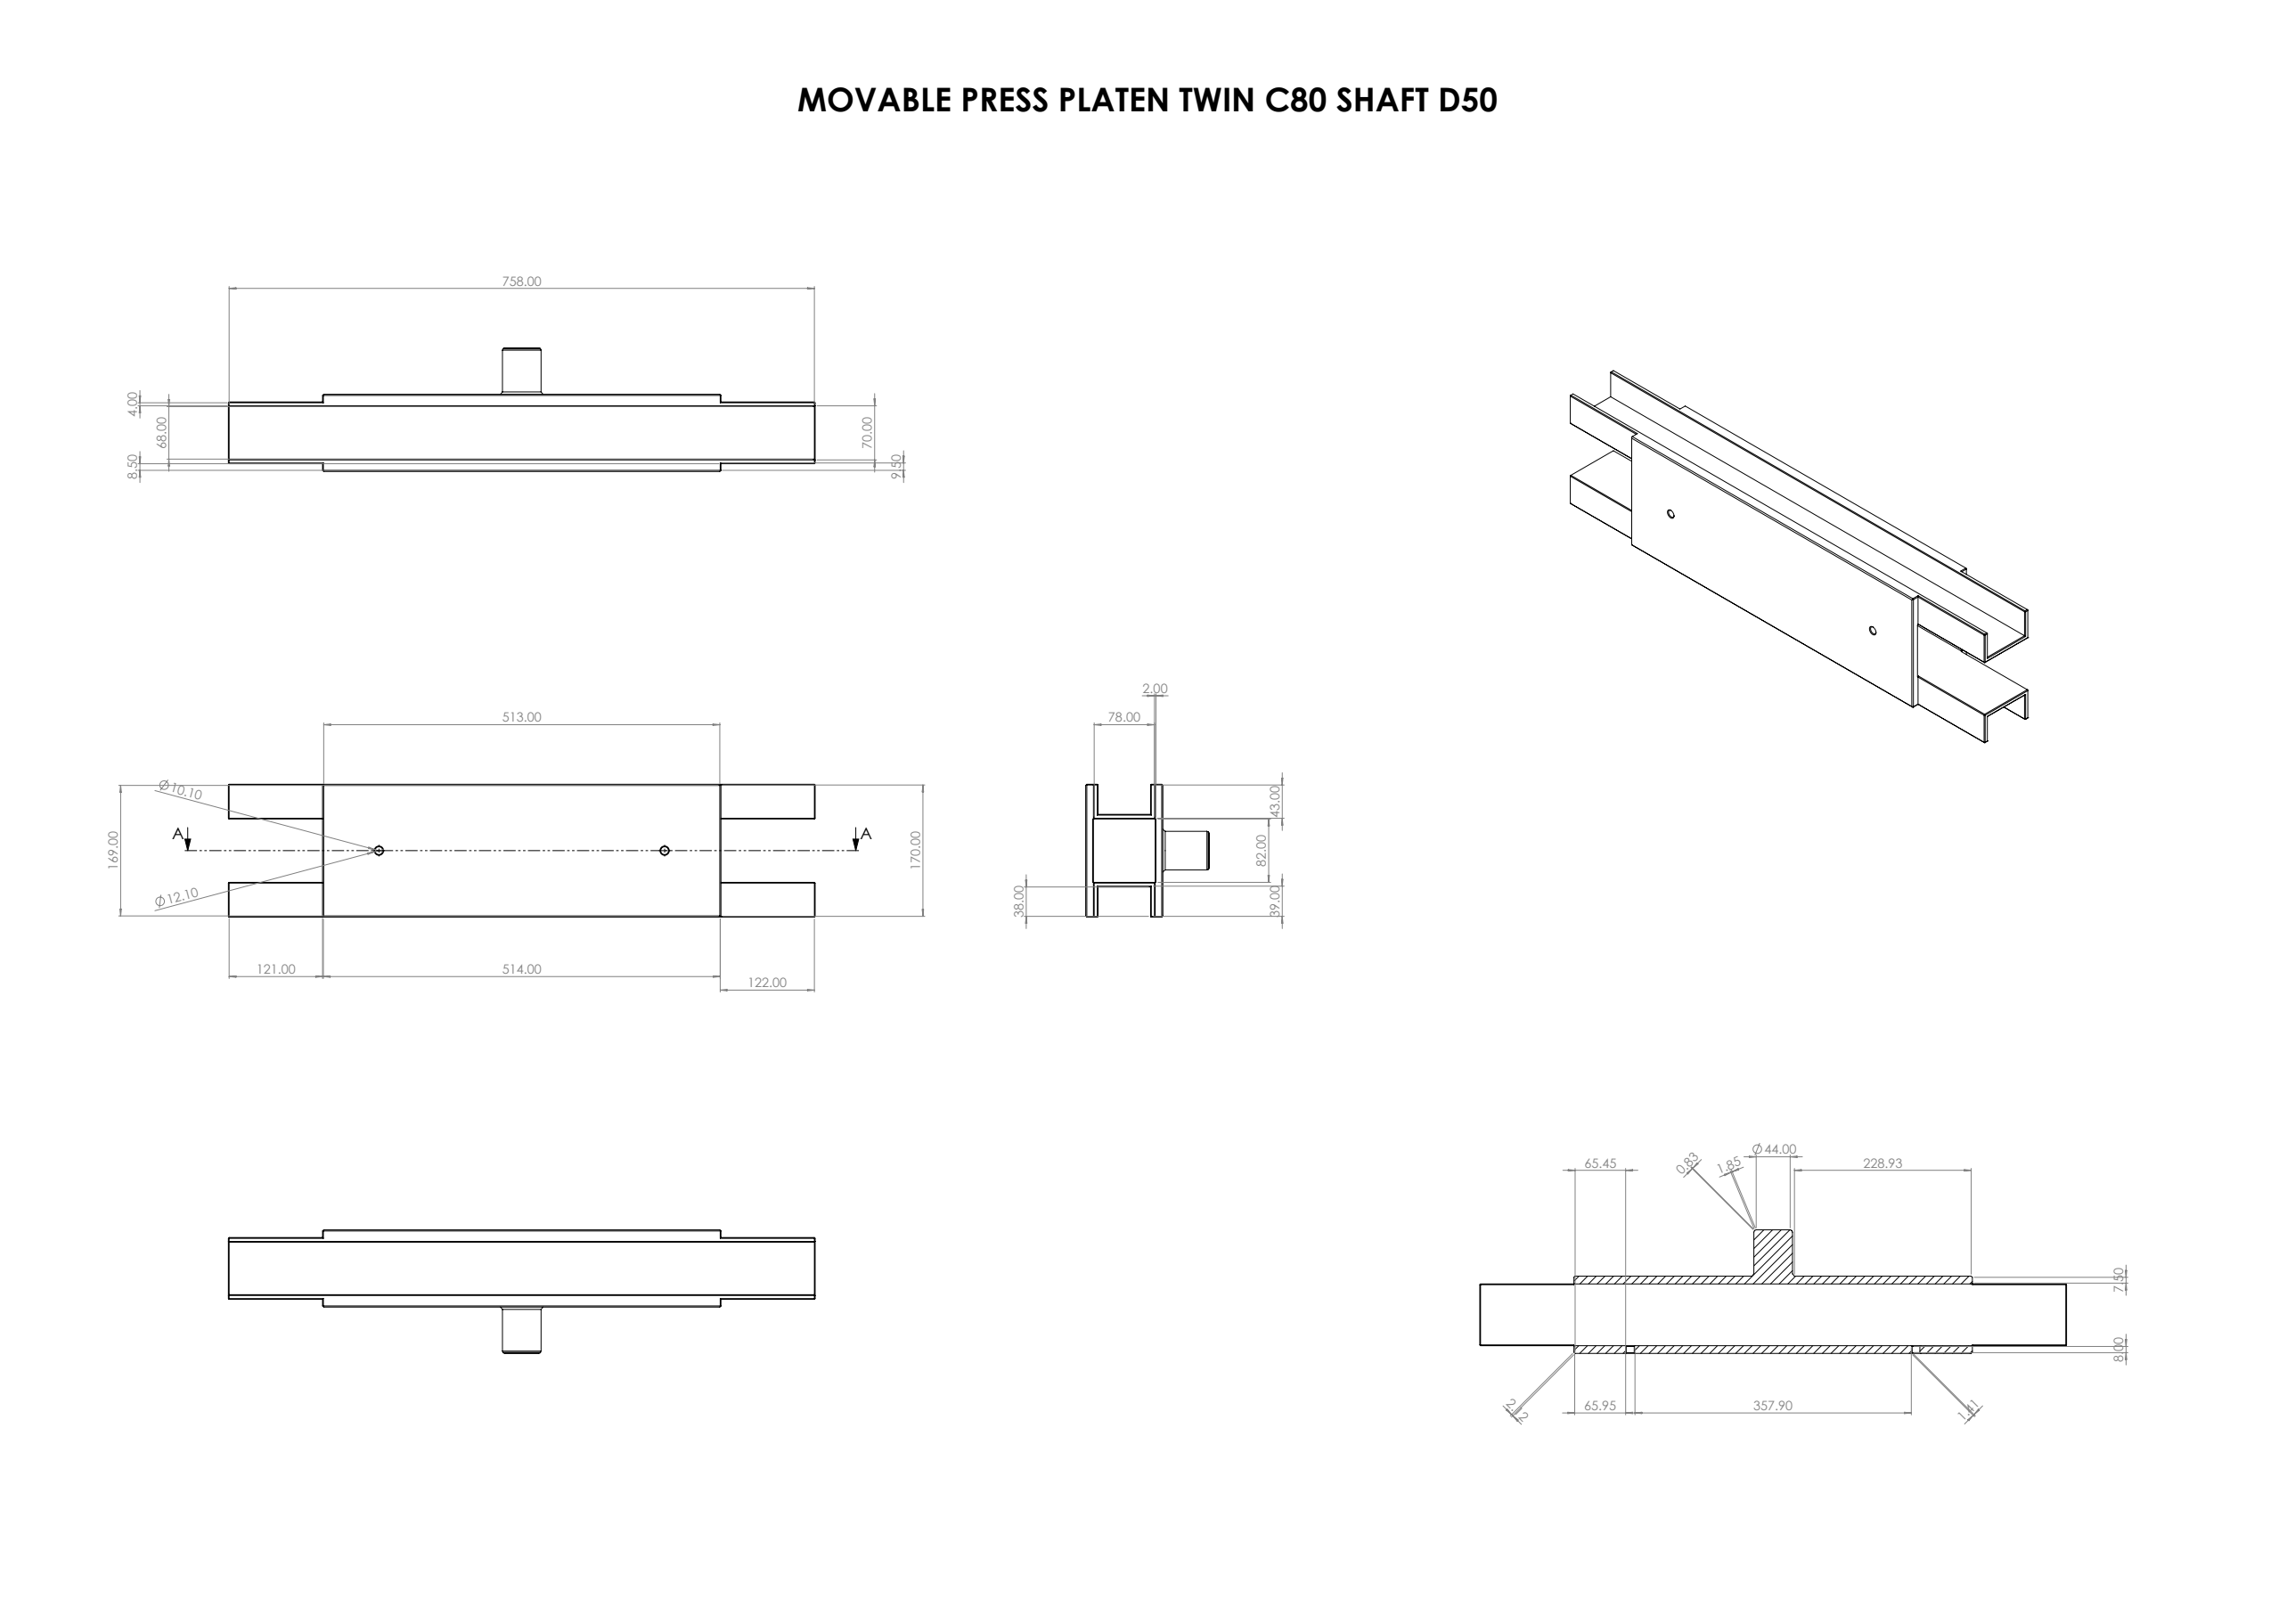
ISO-10303-21;
HEADER;
/* Generated by software containing ST-Developer
 * from STEP Tools, Inc. (www.steptools.com) 
 */

FILE_DESCRIPTION(
/* description */ (''),
/* implementation_level */ '2;1');

FILE_NAME(
/* name */ '03_Movable_Press_Platen_Twin_C80_Shaft_D50.step',
/* time_stamp */ '2026-10-20T10:03:03-07:00',
/* author */ (''),
/* organization */ (''),
/* preprocessor_version */ 'ST-DEVELOPER v20.2',
/* originating_system */ 'Autodesk Translation Framework v15.15.0.0',
/* authorisation */ '');

FILE_SCHEMA (('AUTOMOTIVE_DESIGN { 1 0 10303 214 3 1 1 }'));
ENDSEC;

DATA;
#10=MECHANICAL_DESIGN_GEOMETRIC_PRESENTATION_REPRESENTATION('',(#525),#71492);
#383=SHAPE_REPRESENTATION_RELATIONSHIP('SRR','None',#71604,#402);
#402=ADVANCED_BREP_SHAPE_REPRESENTATION('',(#421),#71474);
#421=MANIFOLD_SOLID_BREP('Platen',#28460);
#525=STYLED_ITEM('',(#71887),#421);
#1566=CYLINDRICAL_SURFACE('',#29155,2.5);
#1567=CYLINDRICAL_SURFACE('',#29162,0.504999999999999);
#1568=CYLINDRICAL_SURFACE('',#29170,0.504999999999999);
#1905=FACE_BOUND('',#4962,.T.);
#1906=FACE_BOUND('',#4963,.T.);
#1907=FACE_BOUND('',#5001,.T.);
#1908=FACE_BOUND('',#5002,.T.);
#1909=FACE_BOUND('',#5010,.T.);
#2197=CIRCLE('',#29117,0.605);
#2198=CIRCLE('',#29118,0.605);
#2199=CIRCLE('',#29148,2.5);
#2200=CIRCLE('',#29149,2.5);
#2201=CIRCLE('',#29150,2.42928932188135);
#2202=CIRCLE('',#29151,2.42928932188135);
#2203=CIRCLE('',#29153,2.37071067811866);
#2204=CIRCLE('',#29154,2.37071067811866);
#2205=CIRCLE('',#29156,2.5);
#2206=CIRCLE('',#29158,2.2);
#2207=CIRCLE('',#29161,0.504999999999999);
#2208=CIRCLE('',#29163,0.504999999999999);
#2209=CIRCLE('',#29165,0.605);
#2210=CIRCLE('',#29167,0.605);
#2211=CIRCLE('',#29169,0.504999999999999);
#2212=CIRCLE('',#29171,0.504999999999999);
#2213=CIRCLE('',#29174,2.75714285714286);
#2799=CONICAL_SURFACE('',#29147,2.46464466094067,0.392699081698708);
#2800=CONICAL_SURFACE('',#29152,2.4,0.785398163397442);
#2801=CONICAL_SURFACE('',#29157,2.28535533905933,1.17809724509617);
#2802=CONICAL_SURFACE('',#29160,0.555,0.785398163397484);
#2803=CONICAL_SURFACE('',#29164,0.555,0.785398163397484);
#2804=CONICAL_SURFACE('',#29168,0.555,0.785398163397484);
#2805=CONICAL_SURFACE('',#29172,0.555,0.785398163397484);
#2806=CONICAL_SURFACE('',#29173,2.65,0.708626272127678);
#3280=FACE_OUTER_BOUND('',#4891,.T.);
#3281=FACE_OUTER_BOUND('',#4892,.T.);
#3282=FACE_OUTER_BOUND('',#4893,.T.);
#3283=FACE_OUTER_BOUND('',#4894,.T.);
#3284=FACE_OUTER_BOUND('',#4895,.T.);
#3285=FACE_OUTER_BOUND('',#4896,.T.);
#3286=FACE_OUTER_BOUND('',#4897,.T.);
#3287=FACE_OUTER_BOUND('',#4898,.T.);
#3288=FACE_OUTER_BOUND('',#4899,.T.);
#3289=FACE_OUTER_BOUND('',#4900,.T.);
#3290=FACE_OUTER_BOUND('',#4901,.T.);
#3291=FACE_OUTER_BOUND('',#4902,.T.);
#3292=FACE_OUTER_BOUND('',#4903,.T.);
#3293=FACE_OUTER_BOUND('',#4904,.T.);
#3294=FACE_OUTER_BOUND('',#4905,.T.);
#3295=FACE_OUTER_BOUND('',#4906,.T.);
#3296=FACE_OUTER_BOUND('',#4907,.T.);
#3297=FACE_OUTER_BOUND('',#4908,.T.);
#3298=FACE_OUTER_BOUND('',#4909,.T.);
#3299=FACE_OUTER_BOUND('',#4910,.T.);
#3300=FACE_OUTER_BOUND('',#4911,.T.);
#3301=FACE_OUTER_BOUND('',#4912,.T.);
#3302=FACE_OUTER_BOUND('',#4913,.T.);
#3303=FACE_OUTER_BOUND('',#4914,.T.);
#3304=FACE_OUTER_BOUND('',#4915,.T.);
#3305=FACE_OUTER_BOUND('',#4916,.T.);
#3306=FACE_OUTER_BOUND('',#4917,.T.);
#3307=FACE_OUTER_BOUND('',#4918,.T.);
#3308=FACE_OUTER_BOUND('',#4919,.T.);
#3309=FACE_OUTER_BOUND('',#4920,.T.);
#3310=FACE_OUTER_BOUND('',#4921,.T.);
#3311=FACE_OUTER_BOUND('',#4922,.T.);
#3312=FACE_OUTER_BOUND('',#4923,.T.);
#3313=FACE_OUTER_BOUND('',#4924,.T.);
#3314=FACE_OUTER_BOUND('',#4925,.T.);
#3315=FACE_OUTER_BOUND('',#4926,.T.);
#3316=FACE_OUTER_BOUND('',#4927,.T.);
#3317=FACE_OUTER_BOUND('',#4928,.T.);
#3318=FACE_OUTER_BOUND('',#4929,.T.);
#3319=FACE_OUTER_BOUND('',#4930,.T.);
#3320=FACE_OUTER_BOUND('',#4931,.T.);
#3321=FACE_OUTER_BOUND('',#4932,.T.);
#3322=FACE_OUTER_BOUND('',#4933,.T.);
#3323=FACE_OUTER_BOUND('',#4934,.T.);
#3324=FACE_OUTER_BOUND('',#4935,.T.);
#3325=FACE_OUTER_BOUND('',#4936,.T.);
#3326=FACE_OUTER_BOUND('',#4937,.T.);
#3327=FACE_OUTER_BOUND('',#4938,.T.);
#3328=FACE_OUTER_BOUND('',#4939,.T.);
#3329=FACE_OUTER_BOUND('',#4940,.T.);
#3330=FACE_OUTER_BOUND('',#4941,.T.);
#3331=FACE_OUTER_BOUND('',#4942,.T.);
#3332=FACE_OUTER_BOUND('',#4943,.T.);
#3333=FACE_OUTER_BOUND('',#4944,.T.);
#3334=FACE_OUTER_BOUND('',#4945,.T.);
#3335=FACE_OUTER_BOUND('',#4946,.T.);
#3336=FACE_OUTER_BOUND('',#4947,.T.);
#3337=FACE_OUTER_BOUND('',#4948,.T.);
#3338=FACE_OUTER_BOUND('',#4949,.T.);
#3339=FACE_OUTER_BOUND('',#4950,.T.);
#3340=FACE_OUTER_BOUND('',#4951,.T.);
#3341=FACE_OUTER_BOUND('',#4952,.T.);
#3342=FACE_OUTER_BOUND('',#4953,.T.);
#3343=FACE_OUTER_BOUND('',#4954,.T.);
#3344=FACE_OUTER_BOUND('',#4955,.T.);
#3345=FACE_OUTER_BOUND('',#4956,.T.);
#3346=FACE_OUTER_BOUND('',#4957,.T.);
#3347=FACE_OUTER_BOUND('',#4958,.T.);
#3348=FACE_OUTER_BOUND('',#4959,.T.);
#3349=FACE_OUTER_BOUND('',#4960,.T.);
#3350=FACE_OUTER_BOUND('',#4961,.T.);
#3351=FACE_OUTER_BOUND('',#4964,.T.);
#3352=FACE_OUTER_BOUND('',#4965,.T.);
#3353=FACE_OUTER_BOUND('',#4966,.T.);
#3354=FACE_OUTER_BOUND('',#4967,.T.);
#3355=FACE_OUTER_BOUND('',#4968,.T.);
#3356=FACE_OUTER_BOUND('',#4969,.T.);
#3357=FACE_OUTER_BOUND('',#4970,.T.);
#3358=FACE_OUTER_BOUND('',#4971,.T.);
#3359=FACE_OUTER_BOUND('',#4972,.T.);
#3360=FACE_OUTER_BOUND('',#4973,.T.);
#3361=FACE_OUTER_BOUND('',#4974,.T.);
#3362=FACE_OUTER_BOUND('',#4975,.T.);
#3363=FACE_OUTER_BOUND('',#4976,.T.);
#3364=FACE_OUTER_BOUND('',#4977,.T.);
#3365=FACE_OUTER_BOUND('',#4978,.T.);
#3366=FACE_OUTER_BOUND('',#4979,.T.);
#3367=FACE_OUTER_BOUND('',#4980,.T.);
#3368=FACE_OUTER_BOUND('',#4981,.T.);
#3369=FACE_OUTER_BOUND('',#4982,.T.);
#3370=FACE_OUTER_BOUND('',#4983,.T.);
#3371=FACE_OUTER_BOUND('',#4984,.T.);
#3372=FACE_OUTER_BOUND('',#4985,.T.);
#3373=FACE_OUTER_BOUND('',#4986,.T.);
#3374=FACE_OUTER_BOUND('',#4987,.T.);
#3375=FACE_OUTER_BOUND('',#4988,.T.);
#3376=FACE_OUTER_BOUND('',#4989,.T.);
#3377=FACE_OUTER_BOUND('',#4990,.T.);
#3378=FACE_OUTER_BOUND('',#4991,.T.);
#3379=FACE_OUTER_BOUND('',#4992,.T.);
#3380=FACE_OUTER_BOUND('',#4993,.T.);
#3381=FACE_OUTER_BOUND('',#4994,.T.);
#3382=FACE_OUTER_BOUND('',#4995,.T.);
#3383=FACE_OUTER_BOUND('',#4996,.T.);
#3384=FACE_OUTER_BOUND('',#4997,.T.);
#3385=FACE_OUTER_BOUND('',#4998,.T.);
#3386=FACE_OUTER_BOUND('',#4999,.T.);
#3387=FACE_OUTER_BOUND('',#5000,.T.);
#3388=FACE_OUTER_BOUND('',#5003,.T.);
#3389=FACE_OUTER_BOUND('',#5004,.T.);
#3390=FACE_OUTER_BOUND('',#5005,.T.);
#3391=FACE_OUTER_BOUND('',#5006,.T.);
#3392=FACE_OUTER_BOUND('',#5007,.T.);
#3393=FACE_OUTER_BOUND('',#5008,.T.);
#3394=FACE_OUTER_BOUND('',#5009,.T.);
#3395=FACE_OUTER_BOUND('',#5011,.T.);
#3396=FACE_OUTER_BOUND('',#5012,.T.);
#3397=FACE_OUTER_BOUND('',#5013,.T.);
#4891=EDGE_LOOP('',(#19603,#19604,#19605,#19606));
#4892=EDGE_LOOP('',(#19607,#19608,#19609,#19610,#19611));
#4893=EDGE_LOOP('',(#19612,#19613,#19614,#19615));
#4894=EDGE_LOOP('',(#19616,#19617,#19618,#19619));
#4895=EDGE_LOOP('',(#19620,#19621,#19622,#19623,#19624,#19625));
#4896=EDGE_LOOP('',(#19626,#19627,#19628,#19629,#19630));
#4897=EDGE_LOOP('',(#19631,#19632,#19633,#19634));
#4898=EDGE_LOOP('',(#19635,#19636,#19637,#19638,#19639));
#4899=EDGE_LOOP('',(#19640,#19641,#19642,#19643,#19644,#19645));
#4900=EDGE_LOOP('',(#19646,#19647,#19648,#19649));
#4901=EDGE_LOOP('',(#19650,#19651,#19652,#19653));
#4902=EDGE_LOOP('',(#19654,#19655,#19656,#19657));
#4903=EDGE_LOOP('',(#19658,#19659,#19660,#19661,#19662,#19663));
#4904=EDGE_LOOP('',(#19664,#19665,#19666,#19667,#19668,#19669));
#4905=EDGE_LOOP('',(#19670,#19671,#19672,#19673,#19674));
#4906=EDGE_LOOP('',(#19675,#19676,#19677,#19678,#19679,#19680));
#4907=EDGE_LOOP('',(#19681,#19682,#19683,#19684,#19685,#19686,#19687,#19688));
#4908=EDGE_LOOP('',(#19689,#19690,#19691,#19692,#19693));
#4909=EDGE_LOOP('',(#19694,#19695,#19696,#19697,#19698));
#4910=EDGE_LOOP('',(#19699,#19700,#19701,#19702,#19703,#19704,#19705,#19706));
#4911=EDGE_LOOP('',(#19707,#19708,#19709,#19710,#19711,#19712));
#4912=EDGE_LOOP('',(#19713,#19714,#19715,#19716,#19717,#19718));
#4913=EDGE_LOOP('',(#19719,#19720,#19721,#19722,#19723));
#4914=EDGE_LOOP('',(#19724,#19725,#19726,#19727,#19728,#19729));
#4915=EDGE_LOOP('',(#19730,#19731,#19732,#19733,#19734,#19735));
#4916=EDGE_LOOP('',(#19736,#19737,#19738,#19739,#19740));
#4917=EDGE_LOOP('',(#19741,#19742,#19743,#19744,#19745,#19746));
#4918=EDGE_LOOP('',(#19747,#19748,#19749,#19750,#19751,#19752,#19753,#19754));
#4919=EDGE_LOOP('',(#19755,#19756,#19757,#19758,#19759));
#4920=EDGE_LOOP('',(#19760,#19761,#19762,#19763,#19764));
#4921=EDGE_LOOP('',(#19765,#19766,#19767,#19768,#19769));
#4922=EDGE_LOOP('',(#19770,#19771,#19772,#19773));
#4923=EDGE_LOOP('',(#19774,#19775,#19776,#19777,#19778,#19779,#19780,#19781,
#19782,#19783));
#4924=EDGE_LOOP('',(#19784,#19785,#19786,#19787,#19788,#19789));
#4925=EDGE_LOOP('',(#19790,#19791,#19792));
#4926=EDGE_LOOP('',(#19793,#19794,#19795,#19796,#19797));
#4927=EDGE_LOOP('',(#19798,#19799,#19800,#19801));
#4928=EDGE_LOOP('',(#19802,#19803,#19804,#19805,#19806,#19807,#19808,#19809));
#4929=EDGE_LOOP('',(#19810,#19811,#19812,#19813,#19814,#19815));
#4930=EDGE_LOOP('',(#19816,#19817,#19818,#19819,#19820));
#4931=EDGE_LOOP('',(#19821,#19822,#19823,#19824,#19825,#19826,#19827,#19828,
#19829,#19830,#19831,#19832,#19833,#19834,#19835,#19836));
#4932=EDGE_LOOP('',(#19837,#19838,#19839,#19840,#19841));
#4933=EDGE_LOOP('',(#19842,#19843,#19844,#19845,#19846,#19847));
#4934=EDGE_LOOP('',(#19848,#19849,#19850,#19851,#19852,#19853));
#4935=EDGE_LOOP('',(#19854,#19855,#19856,#19857,#19858));
#4936=EDGE_LOOP('',(#19859,#19860,#19861,#19862,#19863));
#4937=EDGE_LOOP('',(#19864,#19865,#19866,#19867,#19868,#19869));
#4938=EDGE_LOOP('',(#19870,#19871,#19872,#19873,#19874,#19875));
#4939=EDGE_LOOP('',(#19876,#19877,#19878,#19879));
#4940=EDGE_LOOP('',(#19880,#19881,#19882,#19883,#19884,#19885,#19886,#19887,
#19888,#19889));
#4941=EDGE_LOOP('',(#19890,#19891,#19892,#19893,#19894));
#4942=EDGE_LOOP('',(#19895,#19896,#19897,#19898,#19899,#19900));
#4943=EDGE_LOOP('',(#19901,#19902,#19903,#19904,#19905));
#4944=EDGE_LOOP('',(#19906,#19907,#19908,#19909));
#4945=EDGE_LOOP('',(#19910,#19911,#19912,#19913,#19914));
#4946=EDGE_LOOP('',(#19915,#19916,#19917,#19918,#19919,#19920,#19921,#19922));
#4947=EDGE_LOOP('',(#19923,#19924,#19925,#19926,#19927,#19928));
#4948=EDGE_LOOP('',(#19929,#19930,#19931,#19932));
#4949=EDGE_LOOP('',(#19933,#19934,#19935,#19936));
#4950=EDGE_LOOP('',(#19937,#19938,#19939,#19940,#19941));
#4951=EDGE_LOOP('',(#19942,#19943,#19944,#19945,#19946,#19947,#19948,#19949));
#4952=EDGE_LOOP('',(#19950,#19951,#19952,#19953,#19954));
#4953=EDGE_LOOP('',(#19955,#19956,#19957,#19958,#19959,#19960));
#4954=EDGE_LOOP('',(#19961,#19962,#19963,#19964,#19965));
#4955=EDGE_LOOP('',(#19966,#19967,#19968,#19969,#19970));
#4956=EDGE_LOOP('',(#19971,#19972,#19973,#19974));
#4957=EDGE_LOOP('',(#19975,#19976,#19977,#19978,#19979));
#4958=EDGE_LOOP('',(#19980,#19981,#19982,#19983));
#4959=EDGE_LOOP('',(#19984,#19985,#19986,#19987,#19988,#19989,#19990,#19991,
#19992,#19993));
#4960=EDGE_LOOP('',(#19994,#19995,#19996,#19997));
#4961=EDGE_LOOP('',(#19998,#19999,#20000,#20001));
#4962=EDGE_LOOP('',(#20002));
#4963=EDGE_LOOP('',(#20003));
#4964=EDGE_LOOP('',(#20004,#20005,#20006,#20007,#20008));
#4965=EDGE_LOOP('',(#20009,#20010,#20011,#20012,#20013,#20014,#20015,#20016,
#20017,#20018,#20019,#20020,#20021,#20022,#20023,#20024));
#4966=EDGE_LOOP('',(#20025,#20026,#20027,#20028,#20029));
#4967=EDGE_LOOP('',(#20030,#20031,#20032,#20033,#20034,#20035));
#4968=EDGE_LOOP('',(#20036,#20037,#20038,#20039,#20040,#20041));
#4969=EDGE_LOOP('',(#20042,#20043,#20044,#20045));
#4970=EDGE_LOOP('',(#20046,#20047,#20048,#20049,#20050,#20051));
#4971=EDGE_LOOP('',(#20052,#20053,#20054,#20055,#20056));
#4972=EDGE_LOOP('',(#20057,#20058,#20059,#20060,#20061));
#4973=EDGE_LOOP('',(#20062,#20063,#20064,#20065,#20066));
#4974=EDGE_LOOP('',(#20067,#20068,#20069,#20070));
#4975=EDGE_LOOP('',(#20071,#20072,#20073,#20074,#20075,#20076,#20077,#20078));
#4976=EDGE_LOOP('',(#20079,#20080,#20081,#20082,#20083,#20084));
#4977=EDGE_LOOP('',(#20085,#20086,#20087));
#4978=EDGE_LOOP('',(#20088,#20089,#20090,#20091));
#4979=EDGE_LOOP('',(#20092,#20093,#20094,#20095,#20096));
#4980=EDGE_LOOP('',(#20097,#20098,#20099,#20100));
#4981=EDGE_LOOP('',(#20101,#20102,#20103,#20104,#20105));
#4982=EDGE_LOOP('',(#20106,#20107,#20108,#20109,#20110,#20111));
#4983=EDGE_LOOP('',(#20112,#20113,#20114,#20115,#20116));
#4984=EDGE_LOOP('',(#20117,#20118,#20119,#20120));
#4985=EDGE_LOOP('',(#20121,#20122,#20123,#20124,#20125,#20126,#20127,#20128));
#4986=EDGE_LOOP('',(#20129,#20130,#20131,#20132,#20133));
#4987=EDGE_LOOP('',(#20134,#20135,#20136,#20137,#20138,#20139));
#4988=EDGE_LOOP('',(#20140,#20141,#20142,#20143,#20144,#20145));
#4989=EDGE_LOOP('',(#20146,#20147,#20148,#20149,#20150));
#4990=EDGE_LOOP('',(#20151,#20152,#20153,#20154,#20155,#20156));
#4991=EDGE_LOOP('',(#20157,#20158,#20159,#20160,#20161,#20162));
#4992=EDGE_LOOP('',(#20163,#20164,#20165,#20166,#20167,#20168));
#4993=EDGE_LOOP('',(#20169,#20170,#20171,#20172,#20173,#20174));
#4994=EDGE_LOOP('',(#20175,#20176,#20177,#20178,#20179));
#4995=EDGE_LOOP('',(#20180,#20181,#20182,#20183,#20184));
#4996=EDGE_LOOP('',(#20185));
#4997=EDGE_LOOP('',(#20186,#20187,#20188,#20189));
#4998=EDGE_LOOP('',(#20190,#20191,#20192,#20193));
#4999=EDGE_LOOP('',(#20194,#20195,#20196,#20197));
#5000=EDGE_LOOP('',(#20198,#20199,#20200,#20201));
#5001=EDGE_LOOP('',(#20202));
#5002=EDGE_LOOP('',(#20203));
#5003=EDGE_LOOP('',(#20204,#20205,#20206,#20207));
#5004=EDGE_LOOP('',(#20208,#20209,#20210,#20211));
#5005=EDGE_LOOP('',(#20212,#20213,#20214,#20215));
#5006=EDGE_LOOP('',(#20216,#20217,#20218,#20219));
#5007=EDGE_LOOP('',(#20220,#20221,#20222,#20223));
#5008=EDGE_LOOP('',(#20224,#20225,#20226,#20227));
#5009=EDGE_LOOP('',(#20228,#20229,#20230,#20231));
#5010=EDGE_LOOP('',(#20232));
#5011=EDGE_LOOP('',(#20233,#20234,#20235,#20236));
#5012=EDGE_LOOP('',(#20237,#20238,#20239,#20240,#20241,#20242,#20243,#20244,
#20245,#20246));
#5013=EDGE_LOOP('',(#20247,#20248,#20249,#20250));
#6758=LINE('',#42157,#9246);
#6759=LINE('',#42159,#9247);
#6760=LINE('',#42161,#9248);
#6761=LINE('',#42162,#9249);
#6762=LINE('',#42165,#9250);
#6763=LINE('',#42167,#9251);
#6764=LINE('',#42169,#9252);
#6765=LINE('',#42170,#9253);
#6766=LINE('',#42173,#9254);
#6767=LINE('',#42175,#9255);
#6768=LINE('',#42176,#9256);
#6769=LINE('',#42179,#9257);
#6770=LINE('',#42180,#9258);
#6771=LINE('',#42183,#9259);
#6772=LINE('',#42185,#9260);
#6773=LINE('',#42187,#9261);
#6774=LINE('',#42188,#9262);
#6775=LINE('',#42192,#9263);
#6776=LINE('',#42194,#9264);
#6777=LINE('',#42196,#9265);
#6778=LINE('',#42198,#9266);
#6779=LINE('',#42199,#9267);
#6780=LINE('',#42202,#9268);
#6781=LINE('',#42204,#9269);
#6782=LINE('',#42205,#9270);
#6783=LINE('',#42208,#9271);
#6784=LINE('',#42210,#9272);
#6785=LINE('',#42212,#9273);
#6786=LINE('',#42213,#9274);
#6787=LINE('',#42216,#9275);
#6788=LINE('',#42218,#9276);
#6789=LINE('',#42220,#9277);
#6790=LINE('',#42222,#9278);
#6791=LINE('',#42223,#9279);
#6792=LINE('',#42226,#9280);
#6793=LINE('',#42227,#9281);
#6794=LINE('',#42230,#9282);
#6795=LINE('',#42231,#9283);
#6796=LINE('',#42234,#9284);
#6797=LINE('',#42235,#9285);
#6798=LINE('',#42238,#9286);
#6799=LINE('',#42240,#9287);
#6800=LINE('',#42242,#9288);
#6801=LINE('',#42243,#9289);
#6802=LINE('',#42247,#9290);
#6803=LINE('',#42249,#9291);
#6804=LINE('',#42251,#9292);
#6805=LINE('',#42253,#9293);
#6806=LINE('',#42255,#9294);
#6807=LINE('',#42256,#9295);
#6808=LINE('',#42259,#9296);
#6809=LINE('',#42261,#9297);
#6810=LINE('',#42263,#9298);
#6811=LINE('',#42264,#9299);
#6812=LINE('',#42267,#9300);
#6813=LINE('',#42269,#9301);
#6814=LINE('',#42271,#9302);
#6815=LINE('',#42272,#9303);
#6816=LINE('',#42274,#9304);
#6817=LINE('',#42276,#9305);
#6818=LINE('',#42278,#9306);
#6819=LINE('',#42279,#9307);
#6820=LINE('',#42283,#9308);
#6821=LINE('',#42285,#9309);
#6822=LINE('',#42287,#9310);
#6823=LINE('',#42289,#9311);
#6824=LINE('',#42290,#9312);
#6825=LINE('',#42293,#9313);
#6826=LINE('',#42295,#9314);
#6827=LINE('',#42297,#9315);
#6828=LINE('',#42298,#9316);
#6829=LINE('',#42301,#9317);
#6830=LINE('',#42302,#9318);
#6831=LINE('',#42304,#9319);
#6832=LINE('',#42305,#9320);
#6833=LINE('',#42308,#9321);
#6834=LINE('',#42310,#9322);
#6835=LINE('',#42312,#9323);
#6836=LINE('',#42313,#9324);
#6837=LINE('',#42316,#9325);
#6838=LINE('',#42318,#9326);
#6839=LINE('',#42320,#9327);
#6840=LINE('',#42321,#9328);
#6841=LINE('',#42324,#9329);
#6842=LINE('',#42325,#9330);
#6843=LINE('',#42328,#9331);
#6844=LINE('',#42330,#9332);
#6845=LINE('',#42331,#9333);
#6846=LINE('',#42334,#9334);
#6847=LINE('',#42336,#9335);
#6848=LINE('',#42337,#9336);
#6849=LINE('',#42339,#9337);
#6850=LINE('',#42341,#9338);
#6851=LINE('',#42342,#9339);
#6852=LINE('',#42345,#9340);
#6853=LINE('',#42347,#9341);
#6854=LINE('',#42349,#9342);
#6855=LINE('',#42350,#9343);
#6856=LINE('',#42353,#9344);
#6857=LINE('',#42355,#9345);
#6858=LINE('',#42357,#9346);
#6859=LINE('',#42359,#9347);
#6860=LINE('',#42361,#9348);
#6861=LINE('',#42362,#9349);
#6862=LINE('',#42365,#9350);
#6863=LINE('',#42367,#9351);
#6864=LINE('',#42368,#9352);
#6865=LINE('',#42371,#9353);
#6866=LINE('',#42373,#9354);
#6867=LINE('',#42374,#9355);
#6868=LINE('',#42377,#9356);
#6869=LINE('',#42378,#9357);
#6870=LINE('',#42381,#9358);
#6871=LINE('',#42382,#9359);
#6872=LINE('',#42385,#9360);
#6873=LINE('',#42387,#9361);
#6874=LINE('',#42389,#9362);
#6875=LINE('',#42391,#9363);
#6876=LINE('',#42393,#9364);
#6877=LINE('',#42395,#9365);
#6878=LINE('',#42397,#9366);
#6879=LINE('',#42398,#9367);
#6880=LINE('',#42401,#9368);
#6881=LINE('',#42403,#9369);
#6882=LINE('',#42404,#9370);
#6883=LINE('',#42407,#9371);
#6884=LINE('',#42408,#9372);
#6885=LINE('',#42412,#9373);
#6886=LINE('',#42413,#9374);
#6887=LINE('',#42415,#9375);
#6888=LINE('',#42416,#9376);
#6889=LINE('',#42420,#9377);
#6890=LINE('',#42421,#9378);
#6891=LINE('',#42422,#9379);
#6892=LINE('',#42425,#9380);
#6893=LINE('',#42426,#9381);
#6894=LINE('',#42429,#9382);
#6895=LINE('',#42431,#9383);
#6896=LINE('',#42433,#9384);
#6897=LINE('',#42434,#9385);
#6898=LINE('',#42436,#9386);
#6899=LINE('',#42437,#9387);
#6900=LINE('',#42440,#9388);
#6901=LINE('',#42442,#9389);
#6902=LINE('',#42444,#9390);
#6903=LINE('',#42446,#9391);
#6904=LINE('',#42448,#9392);
#6905=LINE('',#42450,#9393);
#6906=LINE('',#42452,#9394);
#6907=LINE('',#42454,#9395);
#6908=LINE('',#42456,#9396);
#6909=LINE('',#42458,#9397);
#6910=LINE('',#42460,#9398);
#6911=LINE('',#42461,#9399);
#6912=LINE('',#42465,#9400);
#6913=LINE('',#42467,#9401);
#6914=LINE('',#42468,#9402);
#6915=LINE('',#42469,#9403);
#6916=LINE('',#42472,#9404);
#6917=LINE('',#42474,#9405);
#6918=LINE('',#42476,#9406);
#6919=LINE('',#42478,#9407);
#6920=LINE('',#42479,#9408);
#6921=LINE('',#42482,#9409);
#6922=LINE('',#42484,#9410);
#6923=LINE('',#42485,#9411);
#6924=LINE('',#42488,#9412);
#6925=LINE('',#42490,#9413);
#6926=LINE('',#42492,#9414);
#6927=LINE('',#42493,#9415);
#6928=LINE('',#42496,#9416);
#6929=LINE('',#42498,#9417);
#6930=LINE('',#42499,#9418);
#6931=LINE('',#42502,#9419);
#6932=LINE('',#42504,#9420);
#6933=LINE('',#42505,#9421);
#6934=LINE('',#42508,#9422);
#6935=LINE('',#42510,#9423);
#6936=LINE('',#42512,#9424);
#6937=LINE('',#42513,#9425);
#6938=LINE('',#42517,#9426);
#6939=LINE('',#42518,#9427);
#6940=LINE('',#42519,#9428);
#6941=LINE('',#42522,#9429);
#6942=LINE('',#42523,#9430);
#6943=LINE('',#42525,#9431);
#6944=LINE('',#42527,#9432);
#6945=LINE('',#42529,#9433);
#6946=LINE('',#42531,#9434);
#6947=LINE('',#42532,#9435);
#6948=LINE('',#42535,#9436);
#6949=LINE('',#42536,#9437);
#6950=LINE('',#42538,#9438);
#6951=LINE('',#42539,#9439);
#6952=LINE('',#42542,#9440);
#6953=LINE('',#42544,#9441);
#6954=LINE('',#42545,#9442);
#6955=LINE('',#42548,#9443);
#6956=LINE('',#42549,#9444);
#6957=LINE('',#42551,#9445);
#6958=LINE('',#42553,#9446);
#6959=LINE('',#42556,#9447);
#6960=LINE('',#42557,#9448);
#6961=LINE('',#42561,#9449);
#6962=LINE('',#42562,#9450);
#6963=LINE('',#42565,#9451);
#6964=LINE('',#42566,#9452);
#6965=LINE('',#42569,#9453);
#6966=LINE('',#42571,#9454);
#6967=LINE('',#42573,#9455);
#6968=LINE('',#42575,#9456);
#6969=LINE('',#42576,#9457);
#6970=LINE('',#42578,#9458);
#6971=LINE('',#42579,#9459);
#6972=LINE('',#42581,#9460);
#6973=LINE('',#42582,#9461);
#6974=LINE('',#42584,#9462);
#6975=LINE('',#42586,#9463);
#6976=LINE('',#42587,#9464);
#6977=LINE('',#42591,#9465);
#6978=LINE('',#42592,#9466);
#6979=LINE('',#42595,#9467);
#6980=LINE('',#42597,#9468);
#6981=LINE('',#42598,#9469);
#6982=LINE('',#42601,#9470);
#6983=LINE('',#42603,#9471);
#6984=LINE('',#42605,#9472);
#6985=LINE('',#42607,#9473);
#6986=LINE('',#42608,#9474);
#6987=LINE('',#42609,#9475);
#6988=LINE('',#42612,#9476);
#6989=LINE('',#42614,#9477);
#6990=LINE('',#42615,#9478);
#6991=LINE('',#42618,#9479);
#6992=LINE('',#42619,#9480);
#6993=LINE('',#42627,#9481);
#6994=LINE('',#42629,#9482);
#6995=LINE('',#42631,#9483);
#6996=LINE('',#42633,#9484);
#6997=LINE('',#42634,#9485);
#6998=LINE('',#42636,#9486);
#6999=LINE('',#42638,#9487);
#7000=LINE('',#42639,#9488);
#7001=LINE('',#42640,#9489);
#7002=LINE('',#42642,#9490);
#7003=LINE('',#42644,#9491);
#7004=LINE('',#42645,#9492);
#7005=LINE('',#42646,#9493);
#7006=LINE('',#42649,#9494);
#7007=LINE('',#42651,#9495);
#7008=LINE('',#42652,#9496);
#7009=LINE('',#42654,#9497);
#7010=LINE('',#42655,#9498);
#7011=LINE('',#42659,#9499);
#7012=LINE('',#42661,#9500);
#7013=LINE('',#42662,#9501);
#7014=LINE('',#42666,#9502);
#7015=LINE('',#42667,#9503);
#7016=LINE('',#42670,#9504);
#7017=LINE('',#42672,#9505);
#7018=LINE('',#42673,#9506);
#7019=LINE('',#42675,#9507);
#7020=LINE('',#42678,#9508);
#7021=LINE('',#42679,#9509);
#7022=LINE('',#42682,#9510);
#7023=LINE('',#42684,#9511);
#7024=LINE('',#42685,#9512);
#7025=LINE('',#42688,#9513);
#7026=LINE('',#42689,#9514);
#7027=LINE('',#42691,#9515);
#7028=LINE('',#42694,#9516);
#7029=LINE('',#42695,#9517);
#7030=LINE('',#42697,#9518);
#7031=LINE('',#42700,#9519);
#7032=LINE('',#42701,#9520);
#7033=LINE('',#42704,#9521);
#7034=LINE('',#42706,#9522);
#7035=LINE('',#42707,#9523);
#7036=LINE('',#42709,#9524);
#7037=LINE('',#42711,#9525);
#7038=LINE('',#42713,#9526);
#7039=LINE('',#42714,#9527);
#7040=LINE('',#42717,#9528);
#7041=LINE('',#42719,#9529);
#7042=LINE('',#42721,#9530);
#7043=LINE('',#42722,#9531);
#7044=LINE('',#42725,#9532);
#7045=LINE('',#42726,#9533);
#7046=LINE('',#42729,#9534);
#7047=LINE('',#42730,#9535);
#7048=LINE('',#42733,#9536);
#7049=LINE('',#42735,#9537);
#7050=LINE('',#42736,#9538);
#7051=LINE('',#42738,#9539);
#7052=LINE('',#42740,#9540);
#7053=LINE('',#42748,#9541);
#7054=LINE('',#42754,#9542);
#7055=LINE('',#42761,#9543);
#7056=LINE('',#42764,#9544);
#7057=LINE('',#42769,#9545);
#7058=LINE('',#42773,#9546);
#7059=LINE('',#42778,#9547);
#7060=LINE('',#42784,#9548);
#7061=LINE('',#42788,#9549);
#7062=LINE('',#42791,#9550);
#7063=LINE('',#42795,#9551);
#7064=LINE('',#42801,#9552);
#9246=VECTOR('',#32029,1.);
#9247=VECTOR('',#32030,1.);
#9248=VECTOR('',#32031,1.);
#9249=VECTOR('',#32032,1.);
#9250=VECTOR('',#32035,1.);
#9251=VECTOR('',#32036,1.);
#9252=VECTOR('',#32037,1.);
#9253=VECTOR('',#32038,1.);
#9254=VECTOR('',#32041,1.);
#9255=VECTOR('',#32042,1.);
#9256=VECTOR('',#32043,1.);
#9257=VECTOR('',#32046,1.);
#9258=VECTOR('',#32047,1.);
#9259=VECTOR('',#32050,1.);
#9260=VECTOR('',#32051,1.);
#9261=VECTOR('',#32052,1.);
#9262=VECTOR('',#32053,1.);
#9263=VECTOR('',#32056,1.);
#9264=VECTOR('',#32057,1.);
#9265=VECTOR('',#32058,1.);
#9266=VECTOR('',#32059,1.);
#9267=VECTOR('',#32060,1.);
#9268=VECTOR('',#32063,1.);
#9269=VECTOR('',#32064,1.);
#9270=VECTOR('',#32065,1.);
#9271=VECTOR('',#32068,1.);
#9272=VECTOR('',#32069,1.);
#9273=VECTOR('',#32070,1.);
#9274=VECTOR('',#32071,1.);
#9275=VECTOR('',#32074,1.);
#9276=VECTOR('',#32075,1.);
#9277=VECTOR('',#32076,1.);
#9278=VECTOR('',#32077,1.);
#9279=VECTOR('',#32078,1.);
#9280=VECTOR('',#32081,1.);
#9281=VECTOR('',#32082,1.);
#9282=VECTOR('',#32085,1.);
#9283=VECTOR('',#32086,1.);
#9284=VECTOR('',#32089,1.);
#9285=VECTOR('',#32090,1.);
#9286=VECTOR('',#32093,1.);
#9287=VECTOR('',#32094,1.);
#9288=VECTOR('',#32095,1.);
#9289=VECTOR('',#32096,1.);
#9290=VECTOR('',#32099,1.);
#9291=VECTOR('',#32100,1.);
#9292=VECTOR('',#32101,1.);
#9293=VECTOR('',#32102,1.);
#9294=VECTOR('',#32103,1.);
#9295=VECTOR('',#32104,1.);
#9296=VECTOR('',#32107,1.);
#9297=VECTOR('',#32108,1.);
#9298=VECTOR('',#32109,1.);
#9299=VECTOR('',#32110,1.);
#9300=VECTOR('',#32113,1.);
#9301=VECTOR('',#32114,1.);
#9302=VECTOR('',#32115,1.);
#9303=VECTOR('',#32116,1.);
#9304=VECTOR('',#32119,1.);
#9305=VECTOR('',#32120,1.);
#9306=VECTOR('',#32121,1.);
#9307=VECTOR('',#32122,1.);
#9308=VECTOR('',#32125,1.);
#9309=VECTOR('',#32126,1.);
#9310=VECTOR('',#32127,1.);
#9311=VECTOR('',#32128,1.);
#9312=VECTOR('',#32129,1.);
#9313=VECTOR('',#32132,1.);
#9314=VECTOR('',#32133,1.);
#9315=VECTOR('',#32134,1.);
#9316=VECTOR('',#32135,1.);
#9317=VECTOR('',#32138,1.);
#9318=VECTOR('',#32139,1.);
#9319=VECTOR('',#32140,1.);
#9320=VECTOR('',#32141,1.);
#9321=VECTOR('',#32144,1.);
#9322=VECTOR('',#32145,1.);
#9323=VECTOR('',#32146,1.);
#9324=VECTOR('',#32147,1.);
#9325=VECTOR('',#32150,1.);
#9326=VECTOR('',#32151,1.);
#9327=VECTOR('',#32152,1.);
#9328=VECTOR('',#32153,1.);
#9329=VECTOR('',#32156,1.);
#9330=VECTOR('',#32157,1.);
#9331=VECTOR('',#32160,1.);
#9332=VECTOR('',#32161,1.);
#9333=VECTOR('',#32162,1.);
#9334=VECTOR('',#32165,1.);
#9335=VECTOR('',#32166,1.);
#9336=VECTOR('',#32167,1.);
#9337=VECTOR('',#32170,1.);
#9338=VECTOR('',#32171,1.);
#9339=VECTOR('',#32172,1.);
#9340=VECTOR('',#32175,1.);
#9341=VECTOR('',#32176,1.);
#9342=VECTOR('',#32177,1.);
#9343=VECTOR('',#32178,1.);
#9344=VECTOR('',#32181,1.);
#9345=VECTOR('',#32182,1.);
#9346=VECTOR('',#32183,1.);
#9347=VECTOR('',#32184,1.);
#9348=VECTOR('',#32185,1.);
#9349=VECTOR('',#32186,1.);
#9350=VECTOR('',#32189,1.);
#9351=VECTOR('',#32190,1.);
#9352=VECTOR('',#32191,1.);
#9353=VECTOR('',#32194,1.);
#9354=VECTOR('',#32195,1.);
#9355=VECTOR('',#32196,1.);
#9356=VECTOR('',#32199,1.);
#9357=VECTOR('',#32200,1.);
#9358=VECTOR('',#32203,1.);
#9359=VECTOR('',#32204,1.);
#9360=VECTOR('',#32207,1.);
#9361=VECTOR('',#32208,1.);
#9362=VECTOR('',#32209,1.);
#9363=VECTOR('',#32210,1.);
#9364=VECTOR('',#32211,1.);
#9365=VECTOR('',#32212,1.);
#9366=VECTOR('',#32213,1.);
#9367=VECTOR('',#32214,1.);
#9368=VECTOR('',#32217,1.);
#9369=VECTOR('',#32218,1.);
#9370=VECTOR('',#32219,1.);
#9371=VECTOR('',#32222,1.);
#9372=VECTOR('',#32223,1.);
#9373=VECTOR('',#32226,1.);
#9374=VECTOR('',#32227,1.);
#9375=VECTOR('',#32228,1.);
#9376=VECTOR('',#32229,1.);
#9377=VECTOR('',#32232,1.);
#9378=VECTOR('',#32233,1.);
#9379=VECTOR('',#32234,1.);
#9380=VECTOR('',#32237,1.);
#9381=VECTOR('',#32238,1.);
#9382=VECTOR('',#32241,1.);
#9383=VECTOR('',#32242,1.);
#9384=VECTOR('',#32243,1.);
#9385=VECTOR('',#32244,1.);
#9386=VECTOR('',#32247,1.);
#9387=VECTOR('',#32248,1.);
#9388=VECTOR('',#32251,1.);
#9389=VECTOR('',#32252,1.);
#9390=VECTOR('',#32253,1.);
#9391=VECTOR('',#32254,1.);
#9392=VECTOR('',#32255,1.);
#9393=VECTOR('',#32256,1.);
#9394=VECTOR('',#32257,1.);
#9395=VECTOR('',#32258,1.);
#9396=VECTOR('',#32259,1.);
#9397=VECTOR('',#32260,1.);
#9398=VECTOR('',#32261,1.);
#9399=VECTOR('',#32262,1.);
#9400=VECTOR('',#32265,1.);
#9401=VECTOR('',#32266,1.);
#9402=VECTOR('',#32267,1.);
#9403=VECTOR('',#32268,1.);
#9404=VECTOR('',#32271,1.);
#9405=VECTOR('',#32272,1.);
#9406=VECTOR('',#32273,1.);
#9407=VECTOR('',#32274,1.);
#9408=VECTOR('',#32275,1.);
#9409=VECTOR('',#32278,1.);
#9410=VECTOR('',#32279,1.);
#9411=VECTOR('',#32280,1.);
#9412=VECTOR('',#32283,1.);
#9413=VECTOR('',#32284,1.);
#9414=VECTOR('',#32285,1.);
#9415=VECTOR('',#32286,1.);
#9416=VECTOR('',#32289,1.);
#9417=VECTOR('',#32290,1.);
#9418=VECTOR('',#32291,1.);
#9419=VECTOR('',#32294,1.);
#9420=VECTOR('',#32295,1.);
#9421=VECTOR('',#32296,1.);
#9422=VECTOR('',#32299,1.);
#9423=VECTOR('',#32300,1.);
#9424=VECTOR('',#32301,1.);
#9425=VECTOR('',#32302,1.);
#9426=VECTOR('',#32305,1.);
#9427=VECTOR('',#32306,1.);
#9428=VECTOR('',#32307,1.);
#9429=VECTOR('',#32310,1.);
#9430=VECTOR('',#32311,1.);
#9431=VECTOR('',#32312,1.);
#9432=VECTOR('',#32313,1.);
#9433=VECTOR('',#32314,1.);
#9434=VECTOR('',#32315,1.);
#9435=VECTOR('',#32316,1.);
#9436=VECTOR('',#32319,1.);
#9437=VECTOR('',#32320,1.);
#9438=VECTOR('',#32323,1.);
#9439=VECTOR('',#32324,1.);
#9440=VECTOR('',#32327,1.);
#9441=VECTOR('',#32328,1.);
#9442=VECTOR('',#32329,1.);
#9443=VECTOR('',#32332,1.);
#9444=VECTOR('',#32333,1.);
#9445=VECTOR('',#32336,1.);
#9446=VECTOR('',#32339,1.);
#9447=VECTOR('',#32342,1.);
#9448=VECTOR('',#32343,1.);
#9449=VECTOR('',#32348,1.);
#9450=VECTOR('',#32349,1.);
#9451=VECTOR('',#32352,1.);
#9452=VECTOR('',#32353,1.);
#9453=VECTOR('',#32356,1.);
#9454=VECTOR('',#32357,1.);
#9455=VECTOR('',#32358,1.);
#9456=VECTOR('',#32359,1.);
#9457=VECTOR('',#32360,1.);
#9458=VECTOR('',#32363,1.);
#9459=VECTOR('',#32364,1.);
#9460=VECTOR('',#32367,1.);
#9461=VECTOR('',#32368,1.);
#9462=VECTOR('',#32371,1.);
#9463=VECTOR('',#32374,1.);
#9464=VECTOR('',#32375,1.);
#9465=VECTOR('',#32380,1.);
#9466=VECTOR('',#32381,1.);
#9467=VECTOR('',#32384,1.);
#9468=VECTOR('',#32385,1.);
#9469=VECTOR('',#32386,1.);
#9470=VECTOR('',#32389,1.);
#9471=VECTOR('',#32390,1.);
#9472=VECTOR('',#32391,1.);
#9473=VECTOR('',#32392,1.);
#9474=VECTOR('',#32393,1.);
#9475=VECTOR('',#32394,1.);
#9476=VECTOR('',#32397,1.);
#9477=VECTOR('',#32398,1.);
#9478=VECTOR('',#32399,1.);
#9479=VECTOR('',#32402,1.);
#9480=VECTOR('',#32403,1.);
#9481=VECTOR('',#32410,1.);
#9482=VECTOR('',#32411,1.);
#9483=VECTOR('',#32412,1.);
#9484=VECTOR('',#32413,1.);
#9485=VECTOR('',#32414,1.);
#9486=VECTOR('',#32417,1.);
#9487=VECTOR('',#32418,1.);
#9488=VECTOR('',#32419,1.);
#9489=VECTOR('',#32420,1.);
#9490=VECTOR('',#32421,1.);
#9491=VECTOR('',#32422,1.);
#9492=VECTOR('',#32423,1.);
#9493=VECTOR('',#32424,1.);
#9494=VECTOR('',#32427,1.);
#9495=VECTOR('',#32428,1.);
#9496=VECTOR('',#32429,1.);
#9497=VECTOR('',#32432,1.);
#9498=VECTOR('',#32433,1.);
#9499=VECTOR('',#32440,1.);
#9500=VECTOR('',#32441,1.);
#9501=VECTOR('',#32442,1.);
#9502=VECTOR('',#32447,1.);
#9503=VECTOR('',#32448,1.);
#9504=VECTOR('',#32451,1.);
#9505=VECTOR('',#32452,1.);
#9506=VECTOR('',#32453,1.);
#9507=VECTOR('',#32456,1.);
#9508=VECTOR('',#32459,1.);
#9509=VECTOR('',#32460,1.);
#9510=VECTOR('',#32463,1.);
#9511=VECTOR('',#32464,1.);
#9512=VECTOR('',#32465,1.);
#9513=VECTOR('',#32468,1.);
#9514=VECTOR('',#32469,1.);
#9515=VECTOR('',#32472,1.);
#9516=VECTOR('',#32475,1.);
#9517=VECTOR('',#32476,1.);
#9518=VECTOR('',#32479,1.);
#9519=VECTOR('',#32482,1.);
#9520=VECTOR('',#32483,1.);
#9521=VECTOR('',#32486,1.);
#9522=VECTOR('',#32487,1.);
#9523=VECTOR('',#32488,1.);
#9524=VECTOR('',#32491,1.);
#9525=VECTOR('',#32492,1.);
#9526=VECTOR('',#32493,1.);
#9527=VECTOR('',#32494,1.);
#9528=VECTOR('',#32499,1.);
#9529=VECTOR('',#32500,1.);
#9530=VECTOR('',#32501,1.);
#9531=VECTOR('',#32502,1.);
#9532=VECTOR('',#32505,1.);
#9533=VECTOR('',#32506,1.);
#9534=VECTOR('',#32509,1.);
#9535=VECTOR('',#32510,1.);
#9536=VECTOR('',#32513,1.);
#9537=VECTOR('',#32514,1.);
#9538=VECTOR('',#32515,1.);
#9539=VECTOR('',#32518,1.);
#9540=VECTOR('',#32521,1.);
#9541=VECTOR('',#32530,2.46464466094067);
#9542=VECTOR('',#32537,2.4);
#9543=VECTOR('',#32546,2.5);
#9544=VECTOR('',#32549,2.28535533905933);
#9545=VECTOR('',#32556,0.555);
#9546=VECTOR('',#32561,0.504999999999999);
#9547=VECTOR('',#32568,0.555);
#9548=VECTOR('',#32575,0.555);
#9549=VECTOR('',#32580,0.504999999999999);
#9550=VECTOR('',#32585,0.555);
#9551=VECTOR('',#32590,2.65);
#9552=VECTOR('',#32601,1.);
#11804=VERTEX_POINT('',#42155);
#11805=VERTEX_POINT('',#42156);
#11806=VERTEX_POINT('',#42158);
#11807=VERTEX_POINT('',#42160);
#11808=VERTEX_POINT('',#42164);
#11809=VERTEX_POINT('',#42166);
#11810=VERTEX_POINT('',#42168);
#11811=VERTEX_POINT('',#42172);
#11812=VERTEX_POINT('',#42174);
#11813=VERTEX_POINT('',#42178);
#11814=VERTEX_POINT('',#42182);
#11815=VERTEX_POINT('',#42184);
#11816=VERTEX_POINT('',#42186);
#11817=VERTEX_POINT('',#42190);
#11818=VERTEX_POINT('',#42191);
#11819=VERTEX_POINT('',#42193);
#11820=VERTEX_POINT('',#42195);
#11821=VERTEX_POINT('',#42197);
#11822=VERTEX_POINT('',#42201);
#11823=VERTEX_POINT('',#42203);
#11824=VERTEX_POINT('',#42207);
#11825=VERTEX_POINT('',#42209);
#11826=VERTEX_POINT('',#42211);
#11827=VERTEX_POINT('',#42215);
#11828=VERTEX_POINT('',#42217);
#11829=VERTEX_POINT('',#42219);
#11830=VERTEX_POINT('',#42221);
#11831=VERTEX_POINT('',#42225);
#11832=VERTEX_POINT('',#42229);
#11833=VERTEX_POINT('',#42233);
#11834=VERTEX_POINT('',#42237);
#11835=VERTEX_POINT('',#42239);
#11836=VERTEX_POINT('',#42241);
#11837=VERTEX_POINT('',#42245);
#11838=VERTEX_POINT('',#42246);
#11839=VERTEX_POINT('',#42248);
#11840=VERTEX_POINT('',#42250);
#11841=VERTEX_POINT('',#42252);
#11842=VERTEX_POINT('',#42254);
#11843=VERTEX_POINT('',#42258);
#11844=VERTEX_POINT('',#42260);
#11845=VERTEX_POINT('',#42262);
#11846=VERTEX_POINT('',#42266);
#11847=VERTEX_POINT('',#42268);
#11848=VERTEX_POINT('',#42270);
#11849=VERTEX_POINT('',#42275);
#11850=VERTEX_POINT('',#42277);
#11851=VERTEX_POINT('',#42281);
#11852=VERTEX_POINT('',#42282);
#11853=VERTEX_POINT('',#42284);
#11854=VERTEX_POINT('',#42286);
#11855=VERTEX_POINT('',#42288);
#11856=VERTEX_POINT('',#42292);
#11857=VERTEX_POINT('',#42294);
#11858=VERTEX_POINT('',#42296);
#11859=VERTEX_POINT('',#42300);
#11860=VERTEX_POINT('',#42303);
#11861=VERTEX_POINT('',#42307);
#11862=VERTEX_POINT('',#42309);
#11863=VERTEX_POINT('',#42311);
#11864=VERTEX_POINT('',#42315);
#11865=VERTEX_POINT('',#42317);
#11866=VERTEX_POINT('',#42319);
#11867=VERTEX_POINT('',#42323);
#11868=VERTEX_POINT('',#42327);
#11869=VERTEX_POINT('',#42329);
#11870=VERTEX_POINT('',#42333);
#11871=VERTEX_POINT('',#42335);
#11872=VERTEX_POINT('',#42340);
#11873=VERTEX_POINT('',#42344);
#11874=VERTEX_POINT('',#42346);
#11875=VERTEX_POINT('',#42348);
#11876=VERTEX_POINT('',#42352);
#11877=VERTEX_POINT('',#42354);
#11878=VERTEX_POINT('',#42356);
#11879=VERTEX_POINT('',#42358);
#11880=VERTEX_POINT('',#42360);
#11881=VERTEX_POINT('',#42364);
#11882=VERTEX_POINT('',#42366);
#11883=VERTEX_POINT('',#42370);
#11884=VERTEX_POINT('',#42372);
#11885=VERTEX_POINT('',#42376);
#11886=VERTEX_POINT('',#42380);
#11887=VERTEX_POINT('',#42384);
#11888=VERTEX_POINT('',#42386);
#11889=VERTEX_POINT('',#42388);
#11890=VERTEX_POINT('',#42390);
#11891=VERTEX_POINT('',#42392);
#11892=VERTEX_POINT('',#42394);
#11893=VERTEX_POINT('',#42396);
#11894=VERTEX_POINT('',#42400);
#11895=VERTEX_POINT('',#42402);
#11896=VERTEX_POINT('',#42406);
#11897=VERTEX_POINT('',#42410);
#11898=VERTEX_POINT('',#42411);
#11899=VERTEX_POINT('',#42414);
#11900=VERTEX_POINT('',#42418);
#11901=VERTEX_POINT('',#42419);
#11902=VERTEX_POINT('',#42424);
#11903=VERTEX_POINT('',#42428);
#11904=VERTEX_POINT('',#42430);
#11905=VERTEX_POINT('',#42432);
#11906=VERTEX_POINT('',#42439);
#11907=VERTEX_POINT('',#42441);
#11908=VERTEX_POINT('',#42443);
#11909=VERTEX_POINT('',#42445);
#11910=VERTEX_POINT('',#42447);
#11911=VERTEX_POINT('',#42449);
#11912=VERTEX_POINT('',#42451);
#11913=VERTEX_POINT('',#42453);
#11914=VERTEX_POINT('',#42455);
#11915=VERTEX_POINT('',#42457);
#11916=VERTEX_POINT('',#42459);
#11917=VERTEX_POINT('',#42463);
#11918=VERTEX_POINT('',#42464);
#11919=VERTEX_POINT('',#42466);
#11920=VERTEX_POINT('',#42471);
#11921=VERTEX_POINT('',#42473);
#11922=VERTEX_POINT('',#42475);
#11923=VERTEX_POINT('',#42477);
#11924=VERTEX_POINT('',#42481);
#11925=VERTEX_POINT('',#42483);
#11926=VERTEX_POINT('',#42487);
#11927=VERTEX_POINT('',#42489);
#11928=VERTEX_POINT('',#42491);
#11929=VERTEX_POINT('',#42495);
#11930=VERTEX_POINT('',#42497);
#11931=VERTEX_POINT('',#42501);
#11932=VERTEX_POINT('',#42503);
#11933=VERTEX_POINT('',#42507);
#11934=VERTEX_POINT('',#42509);
#11935=VERTEX_POINT('',#42511);
#11936=VERTEX_POINT('',#42515);
#11937=VERTEX_POINT('',#42516);
#11938=VERTEX_POINT('',#42521);
#11939=VERTEX_POINT('',#42524);
#11940=VERTEX_POINT('',#42526);
#11941=VERTEX_POINT('',#42528);
#11942=VERTEX_POINT('',#42530);
#11943=VERTEX_POINT('',#42534);
#11944=VERTEX_POINT('',#42541);
#11945=VERTEX_POINT('',#42543);
#11946=VERTEX_POINT('',#42547);
#11947=VERTEX_POINT('',#42555);
#11948=VERTEX_POINT('',#42560);
#11949=VERTEX_POINT('',#42564);
#11950=VERTEX_POINT('',#42568);
#11951=VERTEX_POINT('',#42570);
#11952=VERTEX_POINT('',#42572);
#11953=VERTEX_POINT('',#42574);
#11954=VERTEX_POINT('',#42590);
#11955=VERTEX_POINT('',#42594);
#11956=VERTEX_POINT('',#42596);
#11957=VERTEX_POINT('',#42600);
#11958=VERTEX_POINT('',#42602);
#11959=VERTEX_POINT('',#42604);
#11960=VERTEX_POINT('',#42606);
#11961=VERTEX_POINT('',#42611);
#11962=VERTEX_POINT('',#42613);
#11963=VERTEX_POINT('',#42617);
#11964=VERTEX_POINT('',#42620);
#11965=VERTEX_POINT('',#42622);
#11966=VERTEX_POINT('',#42625);
#11967=VERTEX_POINT('',#42626);
#11968=VERTEX_POINT('',#42628);
#11969=VERTEX_POINT('',#42630);
#11970=VERTEX_POINT('',#42632);
#11971=VERTEX_POINT('',#42637);
#11972=VERTEX_POINT('',#42641);
#11973=VERTEX_POINT('',#42643);
#11974=VERTEX_POINT('',#42648);
#11975=VERTEX_POINT('',#42650);
#11976=VERTEX_POINT('',#42660);
#11977=VERTEX_POINT('',#42665);
#11978=VERTEX_POINT('',#42669);
#11979=VERTEX_POINT('',#42671);
#11980=VERTEX_POINT('',#42677);
#11981=VERTEX_POINT('',#42681);
#11982=VERTEX_POINT('',#42683);
#11983=VERTEX_POINT('',#42687);
#11984=VERTEX_POINT('',#42693);
#11985=VERTEX_POINT('',#42699);
#11986=VERTEX_POINT('',#42703);
#11987=VERTEX_POINT('',#42705);
#11988=VERTEX_POINT('',#42710);
#11989=VERTEX_POINT('',#42712);
#11990=VERTEX_POINT('',#42718);
#11991=VERTEX_POINT('',#42720);
#11992=VERTEX_POINT('',#42724);
#11993=VERTEX_POINT('',#42728);
#11994=VERTEX_POINT('',#42732);
#11995=VERTEX_POINT('',#42734);
#11996=VERTEX_POINT('',#42743);
#11997=VERTEX_POINT('',#42744);
#11998=VERTEX_POINT('',#42747);
#11999=VERTEX_POINT('',#42749);
#12000=VERTEX_POINT('',#42753);
#12001=VERTEX_POINT('',#42755);
#12002=VERTEX_POINT('',#42759);
#12003=VERTEX_POINT('',#42763);
#12004=VERTEX_POINT('',#42768);
#12005=VERTEX_POINT('',#42772);
#12006=VERTEX_POINT('',#42776);
#12007=VERTEX_POINT('',#42780);
#12008=VERTEX_POINT('',#42783);
#12009=VERTEX_POINT('',#42787);
#12010=VERTEX_POINT('',#42793);
#14685=EDGE_CURVE('',#11804,#11805,#6758,.T.);
#14686=EDGE_CURVE('',#11805,#11806,#6759,.F.);
#14687=EDGE_CURVE('',#11806,#11807,#6760,.T.);
#14688=EDGE_CURVE('',#11807,#11804,#6761,.T.);
#14689=EDGE_CURVE('',#11807,#11808,#6762,.T.);
#14690=EDGE_CURVE('',#11808,#11809,#6763,.T.);
#14691=EDGE_CURVE('',#11809,#11810,#6764,.T.);
#14692=EDGE_CURVE('',#11810,#11804,#6765,.T.);
#14693=EDGE_CURVE('',#11804,#11811,#6766,.T.);
#14694=EDGE_CURVE('',#11812,#11811,#6767,.T.);
#14695=EDGE_CURVE('',#11805,#11812,#6768,.T.);
#14696=EDGE_CURVE('',#11813,#11810,#6769,.T.);
#14697=EDGE_CURVE('',#11811,#11813,#6770,.T.);
#14698=EDGE_CURVE('',#11809,#11814,#6771,.T.);
#14699=EDGE_CURVE('',#11814,#11815,#6772,.T.);
#14700=EDGE_CURVE('',#11815,#11816,#6773,.T.);
#14701=EDGE_CURVE('',#11813,#11816,#6774,.T.);
#14702=EDGE_CURVE('',#11817,#11818,#6775,.T.);
#14703=EDGE_CURVE('',#11818,#11819,#6776,.T.);
#14704=EDGE_CURVE('',#11819,#11820,#6777,.T.);
#14705=EDGE_CURVE('',#11820,#11821,#6778,.T.);
#14706=EDGE_CURVE('',#11821,#11817,#6779,.T.);
#14707=EDGE_CURVE('',#11822,#11817,#6780,.T.);
#14708=EDGE_CURVE('',#11821,#11823,#6781,.T.);
#14709=EDGE_CURVE('',#11823,#11822,#6782,.T.);
#14710=EDGE_CURVE('',#11823,#11824,#6783,.T.);
#14711=EDGE_CURVE('',#11824,#11825,#6784,.T.);
#14712=EDGE_CURVE('',#11825,#11826,#6785,.T.);
#14713=EDGE_CURVE('',#11826,#11822,#6786,.T.);
#14714=EDGE_CURVE('',#11818,#11827,#6787,.T.);
#14715=EDGE_CURVE('',#11827,#11828,#6788,.T.);
#14716=EDGE_CURVE('',#11828,#11829,#6789,.T.);
#14717=EDGE_CURVE('',#11829,#11830,#6790,.T.);
#14718=EDGE_CURVE('',#11830,#11819,#6791,.T.);
#14719=EDGE_CURVE('',#11817,#11831,#6792,.T.);
#14720=EDGE_CURVE('',#11827,#11831,#6793,.T.);
#14721=EDGE_CURVE('',#11822,#11832,#6794,.T.);
#14722=EDGE_CURVE('',#11831,#11832,#6795,.T.);
#14723=EDGE_CURVE('',#11833,#11826,#6796,.T.);
#14724=EDGE_CURVE('',#11832,#11833,#6797,.T.);
#14725=EDGE_CURVE('',#11825,#11834,#6798,.T.);
#14726=EDGE_CURVE('',#11834,#11835,#6799,.T.);
#14727=EDGE_CURVE('',#11835,#11836,#6800,.T.);
#14728=EDGE_CURVE('',#11833,#11836,#6801,.T.);
#14729=EDGE_CURVE('',#11837,#11838,#6802,.T.);
#14730=EDGE_CURVE('',#11838,#11839,#6803,.T.);
#14731=EDGE_CURVE('',#11839,#11840,#6804,.T.);
#14732=EDGE_CURVE('',#11840,#11841,#6805,.T.);
#14733=EDGE_CURVE('',#11841,#11842,#6806,.T.);
#14734=EDGE_CURVE('',#11842,#11837,#6807,.T.);
#14735=EDGE_CURVE('',#11837,#11843,#6808,.T.);
#14736=EDGE_CURVE('',#11843,#11844,#6809,.T.);
#14737=EDGE_CURVE('',#11844,#11845,#6810,.T.);
#14738=EDGE_CURVE('',#11845,#11838,#6811,.T.);
#14739=EDGE_CURVE('',#11842,#11846,#6812,.T.);
#14740=EDGE_CURVE('',#11847,#11846,#6813,.T.);
#14741=EDGE_CURVE('',#11848,#11847,#6814,.T.);
#14742=EDGE_CURVE('',#11848,#11843,#6815,.T.);
#14743=EDGE_CURVE('',#11846,#11806,#6816,.T.);
#14744=EDGE_CURVE('',#11849,#11841,#6817,.T.);
#14745=EDGE_CURVE('',#11850,#11849,#6818,.T.);
#14746=EDGE_CURVE('',#11808,#11850,#6819,.T.);
#14747=EDGE_CURVE('',#11851,#11852,#6820,.T.);
#14748=EDGE_CURVE('',#11852,#11853,#6821,.T.);
#14749=EDGE_CURVE('',#11853,#11854,#6822,.T.);
#14750=EDGE_CURVE('',#11854,#11855,#6823,.T.);
#14751=EDGE_CURVE('',#11855,#11851,#6824,.T.);
#14752=EDGE_CURVE('',#11855,#11856,#6825,.T.);
#14753=EDGE_CURVE('',#11856,#11857,#6826,.T.);
#14754=EDGE_CURVE('',#11857,#11858,#6827,.T.);
#14755=EDGE_CURVE('',#11858,#11851,#6828,.T.);
#14756=EDGE_CURVE('',#11859,#11858,#6829,.T.);
#14757=EDGE_CURVE('',#11844,#11859,#6830,.T.);
#14758=EDGE_CURVE('',#11860,#11848,#6831,.T.);
#14759=EDGE_CURVE('',#11852,#11860,#6832,.T.);
#14760=EDGE_CURVE('',#11861,#11857,#6833,.T.);
#14761=EDGE_CURVE('',#11861,#11862,#6834,.T.);
#14762=EDGE_CURVE('',#11862,#11863,#6835,.T.);
#14763=EDGE_CURVE('',#11859,#11863,#6836,.T.);
#14764=EDGE_CURVE('',#11856,#11864,#6837,.T.);
#14765=EDGE_CURVE('',#11865,#11864,#6838,.T.);
#14766=EDGE_CURVE('',#11866,#11865,#6839,.T.);
#14767=EDGE_CURVE('',#11866,#11861,#6840,.T.);
#14768=EDGE_CURVE('',#11805,#11867,#6841,.T.);
#14769=EDGE_CURVE('',#11867,#11847,#6842,.T.);
#14770=EDGE_CURVE('',#11867,#11868,#6843,.T.);
#14771=EDGE_CURVE('',#11868,#11869,#6844,.T.);
#14772=EDGE_CURVE('',#11869,#11860,#6845,.T.);
#14773=EDGE_CURVE('',#11870,#11869,#6846,.T.);
#14774=EDGE_CURVE('',#11870,#11871,#6847,.T.);
#14775=EDGE_CURVE('',#11853,#11871,#6848,.T.);
#14776=EDGE_CURVE('',#11868,#11812,#6849,.T.);
#14777=EDGE_CURVE('',#11872,#11812,#6850,.T.);
#14778=EDGE_CURVE('',#11872,#11870,#6851,.T.);
#14779=EDGE_CURVE('',#11830,#11873,#6852,.T.);
#14780=EDGE_CURVE('',#11874,#11873,#6853,.T.);
#14781=EDGE_CURVE('',#11875,#11874,#6854,.T.);
#14782=EDGE_CURVE('',#11875,#11820,#6855,.T.);
#14783=EDGE_CURVE('',#11876,#11829,#6856,.T.);
#14784=EDGE_CURVE('',#11877,#11876,#6857,.T.);
#14785=EDGE_CURVE('',#11878,#11877,#6858,.T.);
#14786=EDGE_CURVE('',#11879,#11878,#6859,.T.);
#14787=EDGE_CURVE('',#11880,#11879,#6860,.T.);
#14788=EDGE_CURVE('',#11873,#11880,#6861,.T.);
#14789=EDGE_CURVE('',#11880,#11881,#6862,.F.);
#14790=EDGE_CURVE('',#11881,#11882,#6863,.T.);
#14791=EDGE_CURVE('',#11882,#11874,#6864,.T.);
#14792=EDGE_CURVE('',#11882,#11883,#6865,.T.);
#14793=EDGE_CURVE('',#11883,#11884,#6866,.T.);
#14794=EDGE_CURVE('',#11884,#11875,#6867,.T.);
#14795=EDGE_CURVE('',#11863,#11885,#6868,.T.);
#14796=EDGE_CURVE('',#11885,#11845,#6869,.T.);
#14797=EDGE_CURVE('',#11845,#11886,#6870,.T.);
#14798=EDGE_CURVE('',#11839,#11886,#6871,.T.);
#14799=EDGE_CURVE('',#11887,#11885,#6872,.T.);
#14800=EDGE_CURVE('',#11888,#11887,#6873,.T.);
#14801=EDGE_CURVE('',#11889,#11888,#6874,.T.);
#14802=EDGE_CURVE('',#11890,#11889,#6875,.F.);
#14803=EDGE_CURVE('',#11891,#11890,#6876,.T.);
#14804=EDGE_CURVE('',#11892,#11891,#6877,.T.);
#14805=EDGE_CURVE('',#11892,#11893,#6878,.T.);
#14806=EDGE_CURVE('',#11893,#11886,#6879,.T.);
#14807=EDGE_CURVE('',#11862,#11894,#6880,.T.);
#14808=EDGE_CURVE('',#11894,#11895,#6881,.T.);
#14809=EDGE_CURVE('',#11887,#11895,#6882,.T.);
#14810=EDGE_CURVE('',#11896,#11883,#6883,.T.);
#14811=EDGE_CURVE('',#11884,#11896,#6884,.T.);
#14812=EDGE_CURVE('',#11897,#11898,#6885,.T.);
#14813=EDGE_CURVE('',#11898,#11884,#6886,.T.);
#14814=EDGE_CURVE('',#11896,#11899,#6887,.T.);
#14815=EDGE_CURVE('',#11899,#11897,#6888,.T.);
#14816=EDGE_CURVE('',#11900,#11901,#6889,.F.);
#14817=EDGE_CURVE('',#11901,#11896,#6890,.T.);
#14818=EDGE_CURVE('',#11883,#11900,#6891,.T.);
#14819=EDGE_CURVE('',#11902,#11898,#6892,.T.);
#14820=EDGE_CURVE('',#11824,#11902,#6893,.T.);
#14821=EDGE_CURVE('',#11897,#11903,#6894,.T.);
#14822=EDGE_CURVE('',#11903,#11904,#6895,.T.);
#14823=EDGE_CURVE('',#11905,#11904,#6896,.T.);
#14824=EDGE_CURVE('',#11905,#11902,#6897,.T.);
#14825=EDGE_CURVE('',#11899,#11890,#6898,.T.);
#14826=EDGE_CURVE('',#11889,#11903,#6899,.T.);
#14827=EDGE_CURVE('',#11901,#11906,#6900,.T.);
#14828=EDGE_CURVE('',#11906,#11907,#6901,.T.);
#14829=EDGE_CURVE('',#11907,#11908,#6902,.T.);
#14830=EDGE_CURVE('',#11909,#11908,#6903,.F.);
#14831=EDGE_CURVE('',#11910,#11909,#6904,.T.);
#14832=EDGE_CURVE('',#11911,#11910,#6905,.T.);
#14833=EDGE_CURVE('',#11912,#11911,#6906,.T.);
#14834=EDGE_CURVE('',#11913,#11912,#6907,.T.);
#14835=EDGE_CURVE('',#11913,#11914,#6908,.T.);
#14836=EDGE_CURVE('',#11914,#11915,#6909,.T.);
#14837=EDGE_CURVE('',#11916,#11915,#6910,.T.);
#14838=EDGE_CURVE('',#11891,#11916,#6911,.F.);
#14839=EDGE_CURVE('',#11917,#11918,#6912,.T.);
#14840=EDGE_CURVE('',#11918,#11919,#6913,.T.);
#14841=EDGE_CURVE('',#11919,#11913,#6914,.F.);
#14842=EDGE_CURVE('',#11912,#11917,#6915,.T.);
#14843=EDGE_CURVE('',#11920,#11917,#6916,.T.);
#14844=EDGE_CURVE('',#11920,#11921,#6917,.T.);
#14845=EDGE_CURVE('',#11921,#11922,#6918,.T.);
#14846=EDGE_CURVE('',#11922,#11923,#6919,.T.);
#14847=EDGE_CURVE('',#11923,#11918,#6920,.T.);
#14848=EDGE_CURVE('',#11924,#11911,#6921,.T.);
#14849=EDGE_CURVE('',#11925,#11924,#6922,.T.);
#14850=EDGE_CURVE('',#11925,#11920,#6923,.T.);
#14851=EDGE_CURVE('',#11876,#11926,#6924,.T.);
#14852=EDGE_CURVE('',#11926,#11927,#6925,.T.);
#14853=EDGE_CURVE('',#11927,#11928,#6926,.T.);
#14854=EDGE_CURVE('',#11928,#11877,#6927,.T.);
#14855=EDGE_CURVE('',#11928,#11929,#6928,.T.);
#14856=EDGE_CURVE('',#11929,#11930,#6929,.T.);
#14857=EDGE_CURVE('',#11930,#11878,#6930,.T.);
#14858=EDGE_CURVE('',#11931,#11828,#6931,.T.);
#14859=EDGE_CURVE('',#11931,#11932,#6932,.T.);
#14860=EDGE_CURVE('',#11926,#11932,#6933,.T.);
#14861=EDGE_CURVE('',#11933,#11930,#6934,.T.);
#14862=EDGE_CURVE('',#11933,#11934,#6935,.T.);
#14863=EDGE_CURVE('',#11935,#11934,#6936,.T.);
#14864=EDGE_CURVE('',#11879,#11935,#6937,.T.);
#14865=EDGE_CURVE('',#11936,#11937,#6938,.F.);
#14866=EDGE_CURVE('',#11937,#11909,#6939,.T.);
#14867=EDGE_CURVE('',#11908,#11936,#6940,.T.);
#14868=EDGE_CURVE('',#11938,#11928,#6941,.T.);
#14869=EDGE_CURVE('',#11910,#11938,#6942,.F.);
#14870=EDGE_CURVE('',#11937,#11939,#6943,.T.);
#14871=EDGE_CURVE('',#11939,#11940,#6944,.T.);
#14872=EDGE_CURVE('',#11941,#11940,#6945,.T.);
#14873=EDGE_CURVE('',#11942,#11941,#6946,.T.);
#14874=EDGE_CURVE('',#11929,#11942,#6947,.T.);
#14875=EDGE_CURVE('',#11938,#11943,#6948,.T.);
#14876=EDGE_CURVE('',#11943,#11924,#6949,.T.);
#14877=EDGE_CURVE('',#11932,#11925,#6950,.T.);
#14878=EDGE_CURVE('',#11943,#11927,#6951,.T.);
#14879=EDGE_CURVE('',#11836,#11944,#6952,.T.);
#14880=EDGE_CURVE('',#11944,#11945,#6953,.T.);
#14881=EDGE_CURVE('',#11945,#11832,#6954,.T.);
#14882=EDGE_CURVE('',#11945,#11946,#6955,.T.);
#14883=EDGE_CURVE('',#11946,#11831,#6956,.T.);
#14884=EDGE_CURVE('',#11946,#11931,#6957,.T.);
#14885=EDGE_CURVE('',#11921,#11944,#6958,.T.);
#14886=EDGE_CURVE('',#11835,#11947,#6959,.T.);
#14887=EDGE_CURVE('',#11922,#11947,#6960,.T.);
#14888=EDGE_CURVE('',#11948,#11923,#6961,.T.);
#14889=EDGE_CURVE('',#11948,#11919,#6962,.T.);
#14890=EDGE_CURVE('',#11947,#11949,#6963,.T.);
#14891=EDGE_CURVE('',#11949,#11948,#6964,.T.);
#14892=EDGE_CURVE('',#11950,#11834,#6965,.T.);
#14893=EDGE_CURVE('',#11951,#11950,#6966,.T.);
#14894=EDGE_CURVE('',#11952,#11951,#6967,.T.);
#14895=EDGE_CURVE('',#11953,#11952,#6968,.T.);
#14896=EDGE_CURVE('',#11949,#11953,#6969,.T.);
#14897=EDGE_CURVE('',#11953,#11865,#6970,.T.);
#14898=EDGE_CURVE('',#11864,#11948,#6971,.T.);
#14899=EDGE_CURVE('',#11895,#11952,#6972,.T.);
#14900=EDGE_CURVE('',#11894,#11866,#6973,.T.);
#14901=EDGE_CURVE('',#11951,#11888,#6974,.T.);
#14902=EDGE_CURVE('',#11950,#11905,#6975,.T.);
#14903=EDGE_CURVE('',#11904,#11888,#6976,.T.);
#14904=EDGE_CURVE('',#11935,#11954,#6977,.T.);
#14905=EDGE_CURVE('',#11954,#11881,#6978,.T.);
#14906=EDGE_CURVE('',#11906,#11955,#6979,.T.);
#14907=EDGE_CURVE('',#11955,#11956,#6980,.F.);
#14908=EDGE_CURVE('',#11956,#11907,#6981,.T.);
#14909=EDGE_CURVE('',#11957,#11954,#6982,.T.);
#14910=EDGE_CURVE('',#11958,#11957,#6983,.T.);
#14911=EDGE_CURVE('',#11959,#11958,#6984,.T.);
#14912=EDGE_CURVE('',#11960,#11959,#6985,.F.);
#14913=EDGE_CURVE('',#11960,#11955,#6986,.T.);
#14914=EDGE_CURVE('',#11881,#11900,#6987,.T.);
#14915=EDGE_CURVE('',#11914,#11961,#6988,.T.);
#14916=EDGE_CURVE('',#11961,#11962,#6989,.F.);
#14917=EDGE_CURVE('',#11962,#11915,#6990,.T.);
#14918=EDGE_CURVE('',#11963,#11962,#6991,.T.);
#14919=EDGE_CURVE('',#11916,#11963,#6992,.T.);
#14920=EDGE_CURVE('',#11964,#11964,#2197,.T.);
#14921=EDGE_CURVE('',#11965,#11965,#2198,.T.);
#14922=EDGE_CURVE('',#11966,#11967,#6993,.T.);
#14923=EDGE_CURVE('',#11967,#11968,#6994,.T.);
#14924=EDGE_CURVE('',#11968,#11969,#6995,.F.);
#14925=EDGE_CURVE('',#11969,#11970,#6996,.T.);
#14926=EDGE_CURVE('',#11970,#11966,#6997,.T.);
#14927=EDGE_CURVE('',#11968,#11961,#6998,.T.);
#14928=EDGE_CURVE('',#11971,#11967,#6999,.T.);
#14929=EDGE_CURVE('',#11939,#11971,#7000,.T.);
#14930=EDGE_CURVE('',#11956,#11936,#7001,.T.);
#14931=EDGE_CURVE('',#11972,#11960,#7002,.T.);
#14932=EDGE_CURVE('',#11973,#11972,#7003,.T.);
#14933=EDGE_CURVE('',#11893,#11973,#7004,.T.);
#14934=EDGE_CURVE('',#11963,#11892,#7005,.F.);
#14935=EDGE_CURVE('',#11974,#11966,#7006,.T.);
#14936=EDGE_CURVE('',#11974,#11975,#7007,.T.);
#14937=EDGE_CURVE('',#11975,#11971,#7008,.T.);
#14938=EDGE_CURVE('',#11871,#11974,#7009,.T.);
#14939=EDGE_CURVE('',#11970,#11854,#7010,.T.);
#14940=EDGE_CURVE('',#11840,#11973,#7011,.T.);
#14941=EDGE_CURVE('',#11972,#11976,#7012,.T.);
#14942=EDGE_CURVE('',#11976,#11849,#7013,.T.);
#14943=EDGE_CURVE('',#11959,#11977,#7014,.T.);
#14944=EDGE_CURVE('',#11976,#11977,#7015,.T.);
#14945=EDGE_CURVE('',#11816,#11978,#7016,.T.);
#14946=EDGE_CURVE('',#11978,#11979,#7017,.T.);
#14947=EDGE_CURVE('',#11979,#11811,#7018,.T.);
#14948=EDGE_CURVE('',#11979,#11872,#7019,.T.);
#14949=EDGE_CURVE('',#11980,#11978,#7020,.T.);
#14950=EDGE_CURVE('',#11975,#11980,#7021,.T.);
#14951=EDGE_CURVE('',#11815,#11981,#7022,.T.);
#14952=EDGE_CURVE('',#11982,#11981,#7023,.T.);
#14953=EDGE_CURVE('',#11980,#11982,#7024,.T.);
#14954=EDGE_CURVE('',#11983,#11975,#7025,.T.);
#14955=EDGE_CURVE('',#11971,#11983,#7026,.T.);
#14956=EDGE_CURVE('',#11983,#11940,#7027,.T.);
#14957=EDGE_CURVE('',#11982,#11984,#7028,.T.);
#14958=EDGE_CURVE('',#11984,#11983,#7029,.T.);
#14959=EDGE_CURVE('',#11941,#11984,#7030,.T.);
#14960=EDGE_CURVE('',#11981,#11985,#7031,.T.);
#14961=EDGE_CURVE('',#11985,#11941,#7032,.T.);
#14962=EDGE_CURVE('',#11977,#11986,#7033,.T.);
#14963=EDGE_CURVE('',#11986,#11987,#7034,.T.);
#14964=EDGE_CURVE('',#11987,#11850,#7035,.T.);
#14965=EDGE_CURVE('',#11986,#11958,#7036,.T.);
#14966=EDGE_CURVE('',#11988,#11958,#7037,.T.);
#14967=EDGE_CURVE('',#11988,#11989,#7038,.T.);
#14968=EDGE_CURVE('',#11989,#11987,#7039,.T.);
#14969=EDGE_CURVE('',#11989,#11814,#7040,.T.);
#14970=EDGE_CURVE('',#11990,#11988,#7041,.T.);
#14971=EDGE_CURVE('',#11991,#11990,#7042,.T.);
#14972=EDGE_CURVE('',#11985,#11991,#7043,.T.);
#14973=EDGE_CURVE('',#11991,#11992,#7044,.T.);
#14974=EDGE_CURVE('',#11992,#11942,#7045,.T.);
#14975=EDGE_CURVE('',#11993,#11992,#7046,.T.);
#14976=EDGE_CURVE('',#11993,#11933,#7047,.T.);
#14977=EDGE_CURVE('',#11994,#11990,#7048,.T.);
#14978=EDGE_CURVE('',#11995,#11994,#7049,.T.);
#14979=EDGE_CURVE('',#11995,#11993,#7050,.T.);
#14980=EDGE_CURVE('',#11957,#11994,#7051,.T.);
#14981=EDGE_CURVE('',#11934,#11995,#7052,.T.);
#14982=EDGE_CURVE('',#11996,#11997,#2199,.T.);
#14983=EDGE_CURVE('',#11997,#11996,#2200,.T.);
#14984=EDGE_CURVE('',#11996,#11998,#7053,.T.);
#14985=EDGE_CURVE('',#11998,#11999,#2201,.T.);
#14986=EDGE_CURVE('',#11999,#11998,#2202,.T.);
#14987=EDGE_CURVE('',#11999,#12000,#7054,.T.);
#14988=EDGE_CURVE('',#12001,#12000,#2203,.T.);
#14989=EDGE_CURVE('',#12000,#12001,#2204,.T.);
#14990=EDGE_CURVE('',#12002,#12002,#2205,.T.);
#14991=EDGE_CURVE('',#12002,#11997,#7055,.T.);
#14992=EDGE_CURVE('',#12001,#12003,#7056,.T.);
#14993=EDGE_CURVE('',#12003,#12003,#2206,.T.);
#14994=EDGE_CURVE('',#11965,#12004,#7057,.T.);
#14995=EDGE_CURVE('',#12004,#12004,#2207,.T.);
#14996=EDGE_CURVE('',#12004,#12005,#7058,.T.);
#14997=EDGE_CURVE('',#12005,#12005,#2208,.T.);
#14998=EDGE_CURVE('',#12006,#12006,#2209,.T.);
#14999=EDGE_CURVE('',#12006,#12005,#7059,.T.);
#15000=EDGE_CURVE('',#12007,#12007,#2210,.T.);
#15001=EDGE_CURVE('',#11964,#12008,#7060,.T.);
#15002=EDGE_CURVE('',#12008,#12008,#2211,.T.);
#15003=EDGE_CURVE('',#12008,#12009,#7061,.T.);
#15004=EDGE_CURVE('',#12009,#12009,#2212,.T.);
#15005=EDGE_CURVE('',#12007,#12009,#7062,.T.);
#15006=EDGE_CURVE('',#12010,#12010,#2213,.T.);
#15007=EDGE_CURVE('',#12010,#12002,#7063,.T.);
#15008=EDGE_CURVE('',#11969,#11855,#7064,.T.);
#19603=ORIENTED_EDGE('',*,*,#14685,.T.);
#19604=ORIENTED_EDGE('',*,*,#14686,.T.);
#19605=ORIENTED_EDGE('',*,*,#14687,.T.);
#19606=ORIENTED_EDGE('',*,*,#14688,.T.);
#19607=ORIENTED_EDGE('',*,*,#14689,.T.);
#19608=ORIENTED_EDGE('',*,*,#14690,.T.);
#19609=ORIENTED_EDGE('',*,*,#14691,.T.);
#19610=ORIENTED_EDGE('',*,*,#14692,.T.);
#19611=ORIENTED_EDGE('',*,*,#14688,.F.);
#19612=ORIENTED_EDGE('',*,*,#14685,.F.);
#19613=ORIENTED_EDGE('',*,*,#14693,.T.);
#19614=ORIENTED_EDGE('',*,*,#14694,.F.);
#19615=ORIENTED_EDGE('',*,*,#14695,.F.);
#19616=ORIENTED_EDGE('',*,*,#14692,.F.);
#19617=ORIENTED_EDGE('',*,*,#14696,.F.);
#19618=ORIENTED_EDGE('',*,*,#14697,.F.);
#19619=ORIENTED_EDGE('',*,*,#14693,.F.);
#19620=ORIENTED_EDGE('',*,*,#14691,.F.);
#19621=ORIENTED_EDGE('',*,*,#14698,.T.);
#19622=ORIENTED_EDGE('',*,*,#14699,.T.);
#19623=ORIENTED_EDGE('',*,*,#14700,.T.);
#19624=ORIENTED_EDGE('',*,*,#14701,.F.);
#19625=ORIENTED_EDGE('',*,*,#14696,.T.);
#19626=ORIENTED_EDGE('',*,*,#14702,.T.);
#19627=ORIENTED_EDGE('',*,*,#14703,.T.);
#19628=ORIENTED_EDGE('',*,*,#14704,.T.);
#19629=ORIENTED_EDGE('',*,*,#14705,.T.);
#19630=ORIENTED_EDGE('',*,*,#14706,.T.);
#19631=ORIENTED_EDGE('',*,*,#14707,.T.);
#19632=ORIENTED_EDGE('',*,*,#14706,.F.);
#19633=ORIENTED_EDGE('',*,*,#14708,.T.);
#19634=ORIENTED_EDGE('',*,*,#14709,.T.);
#19635=ORIENTED_EDGE('',*,*,#14710,.T.);
#19636=ORIENTED_EDGE('',*,*,#14711,.T.);
#19637=ORIENTED_EDGE('',*,*,#14712,.T.);
#19638=ORIENTED_EDGE('',*,*,#14713,.T.);
#19639=ORIENTED_EDGE('',*,*,#14709,.F.);
#19640=ORIENTED_EDGE('',*,*,#14703,.F.);
#19641=ORIENTED_EDGE('',*,*,#14714,.T.);
#19642=ORIENTED_EDGE('',*,*,#14715,.T.);
#19643=ORIENTED_EDGE('',*,*,#14716,.T.);
#19644=ORIENTED_EDGE('',*,*,#14717,.T.);
#19645=ORIENTED_EDGE('',*,*,#14718,.T.);
#19646=ORIENTED_EDGE('',*,*,#14702,.F.);
#19647=ORIENTED_EDGE('',*,*,#14719,.T.);
#19648=ORIENTED_EDGE('',*,*,#14720,.F.);
#19649=ORIENTED_EDGE('',*,*,#14714,.F.);
#19650=ORIENTED_EDGE('',*,*,#14707,.F.);
#19651=ORIENTED_EDGE('',*,*,#14721,.T.);
#19652=ORIENTED_EDGE('',*,*,#14722,.F.);
#19653=ORIENTED_EDGE('',*,*,#14719,.F.);
#19654=ORIENTED_EDGE('',*,*,#14713,.F.);
#19655=ORIENTED_EDGE('',*,*,#14723,.F.);
#19656=ORIENTED_EDGE('',*,*,#14724,.F.);
#19657=ORIENTED_EDGE('',*,*,#14721,.F.);
#19658=ORIENTED_EDGE('',*,*,#14712,.F.);
#19659=ORIENTED_EDGE('',*,*,#14725,.T.);
#19660=ORIENTED_EDGE('',*,*,#14726,.T.);
#19661=ORIENTED_EDGE('',*,*,#14727,.T.);
#19662=ORIENTED_EDGE('',*,*,#14728,.F.);
#19663=ORIENTED_EDGE('',*,*,#14723,.T.);
#19664=ORIENTED_EDGE('',*,*,#14729,.T.);
#19665=ORIENTED_EDGE('',*,*,#14730,.T.);
#19666=ORIENTED_EDGE('',*,*,#14731,.T.);
#19667=ORIENTED_EDGE('',*,*,#14732,.T.);
#19668=ORIENTED_EDGE('',*,*,#14733,.T.);
#19669=ORIENTED_EDGE('',*,*,#14734,.T.);
#19670=ORIENTED_EDGE('',*,*,#14729,.F.);
#19671=ORIENTED_EDGE('',*,*,#14735,.T.);
#19672=ORIENTED_EDGE('',*,*,#14736,.T.);
#19673=ORIENTED_EDGE('',*,*,#14737,.T.);
#19674=ORIENTED_EDGE('',*,*,#14738,.T.);
#19675=ORIENTED_EDGE('',*,*,#14734,.F.);
#19676=ORIENTED_EDGE('',*,*,#14739,.T.);
#19677=ORIENTED_EDGE('',*,*,#14740,.F.);
#19678=ORIENTED_EDGE('',*,*,#14741,.F.);
#19679=ORIENTED_EDGE('',*,*,#14742,.T.);
#19680=ORIENTED_EDGE('',*,*,#14735,.F.);
#19681=ORIENTED_EDGE('',*,*,#14743,.F.);
#19682=ORIENTED_EDGE('',*,*,#14739,.F.);
#19683=ORIENTED_EDGE('',*,*,#14733,.F.);
#19684=ORIENTED_EDGE('',*,*,#14744,.F.);
#19685=ORIENTED_EDGE('',*,*,#14745,.F.);
#19686=ORIENTED_EDGE('',*,*,#14746,.F.);
#19687=ORIENTED_EDGE('',*,*,#14689,.F.);
#19688=ORIENTED_EDGE('',*,*,#14687,.F.);
#19689=ORIENTED_EDGE('',*,*,#14747,.T.);
#19690=ORIENTED_EDGE('',*,*,#14748,.T.);
#19691=ORIENTED_EDGE('',*,*,#14749,.T.);
#19692=ORIENTED_EDGE('',*,*,#14750,.T.);
#19693=ORIENTED_EDGE('',*,*,#14751,.T.);
#19694=ORIENTED_EDGE('',*,*,#14752,.T.);
#19695=ORIENTED_EDGE('',*,*,#14753,.T.);
#19696=ORIENTED_EDGE('',*,*,#14754,.T.);
#19697=ORIENTED_EDGE('',*,*,#14755,.T.);
#19698=ORIENTED_EDGE('',*,*,#14751,.F.);
#19699=ORIENTED_EDGE('',*,*,#14747,.F.);
#19700=ORIENTED_EDGE('',*,*,#14755,.F.);
#19701=ORIENTED_EDGE('',*,*,#14756,.F.);
#19702=ORIENTED_EDGE('',*,*,#14757,.F.);
#19703=ORIENTED_EDGE('',*,*,#14736,.F.);
#19704=ORIENTED_EDGE('',*,*,#14742,.F.);
#19705=ORIENTED_EDGE('',*,*,#14758,.F.);
#19706=ORIENTED_EDGE('',*,*,#14759,.F.);
#19707=ORIENTED_EDGE('',*,*,#14754,.F.);
#19708=ORIENTED_EDGE('',*,*,#14760,.F.);
#19709=ORIENTED_EDGE('',*,*,#14761,.T.);
#19710=ORIENTED_EDGE('',*,*,#14762,.T.);
#19711=ORIENTED_EDGE('',*,*,#14763,.F.);
#19712=ORIENTED_EDGE('',*,*,#14756,.T.);
#19713=ORIENTED_EDGE('',*,*,#14753,.F.);
#19714=ORIENTED_EDGE('',*,*,#14764,.T.);
#19715=ORIENTED_EDGE('',*,*,#14765,.F.);
#19716=ORIENTED_EDGE('',*,*,#14766,.F.);
#19717=ORIENTED_EDGE('',*,*,#14767,.T.);
#19718=ORIENTED_EDGE('',*,*,#14760,.T.);
#19719=ORIENTED_EDGE('',*,*,#14740,.T.);
#19720=ORIENTED_EDGE('',*,*,#14743,.T.);
#19721=ORIENTED_EDGE('',*,*,#14686,.F.);
#19722=ORIENTED_EDGE('',*,*,#14768,.T.);
#19723=ORIENTED_EDGE('',*,*,#14769,.T.);
#19724=ORIENTED_EDGE('',*,*,#14769,.F.);
#19725=ORIENTED_EDGE('',*,*,#14770,.T.);
#19726=ORIENTED_EDGE('',*,*,#14771,.T.);
#19727=ORIENTED_EDGE('',*,*,#14772,.T.);
#19728=ORIENTED_EDGE('',*,*,#14758,.T.);
#19729=ORIENTED_EDGE('',*,*,#14741,.T.);
#19730=ORIENTED_EDGE('',*,*,#14748,.F.);
#19731=ORIENTED_EDGE('',*,*,#14759,.T.);
#19732=ORIENTED_EDGE('',*,*,#14772,.F.);
#19733=ORIENTED_EDGE('',*,*,#14773,.F.);
#19734=ORIENTED_EDGE('',*,*,#14774,.T.);
#19735=ORIENTED_EDGE('',*,*,#14775,.F.);
#19736=ORIENTED_EDGE('',*,*,#14771,.F.);
#19737=ORIENTED_EDGE('',*,*,#14776,.T.);
#19738=ORIENTED_EDGE('',*,*,#14777,.F.);
#19739=ORIENTED_EDGE('',*,*,#14778,.T.);
#19740=ORIENTED_EDGE('',*,*,#14773,.T.);
#19741=ORIENTED_EDGE('',*,*,#14704,.F.);
#19742=ORIENTED_EDGE('',*,*,#14718,.F.);
#19743=ORIENTED_EDGE('',*,*,#14779,.T.);
#19744=ORIENTED_EDGE('',*,*,#14780,.F.);
#19745=ORIENTED_EDGE('',*,*,#14781,.F.);
#19746=ORIENTED_EDGE('',*,*,#14782,.T.);
#19747=ORIENTED_EDGE('',*,*,#14717,.F.);
#19748=ORIENTED_EDGE('',*,*,#14783,.F.);
#19749=ORIENTED_EDGE('',*,*,#14784,.F.);
#19750=ORIENTED_EDGE('',*,*,#14785,.F.);
#19751=ORIENTED_EDGE('',*,*,#14786,.F.);
#19752=ORIENTED_EDGE('',*,*,#14787,.F.);
#19753=ORIENTED_EDGE('',*,*,#14788,.F.);
#19754=ORIENTED_EDGE('',*,*,#14779,.F.);
#19755=ORIENTED_EDGE('',*,*,#14780,.T.);
#19756=ORIENTED_EDGE('',*,*,#14788,.T.);
#19757=ORIENTED_EDGE('',*,*,#14789,.T.);
#19758=ORIENTED_EDGE('',*,*,#14790,.T.);
#19759=ORIENTED_EDGE('',*,*,#14791,.T.);
#19760=ORIENTED_EDGE('',*,*,#14791,.F.);
#19761=ORIENTED_EDGE('',*,*,#14792,.T.);
#19762=ORIENTED_EDGE('',*,*,#14793,.T.);
#19763=ORIENTED_EDGE('',*,*,#14794,.T.);
#19764=ORIENTED_EDGE('',*,*,#14781,.T.);
#19765=ORIENTED_EDGE('',*,*,#14757,.T.);
#19766=ORIENTED_EDGE('',*,*,#14763,.T.);
#19767=ORIENTED_EDGE('',*,*,#14795,.T.);
#19768=ORIENTED_EDGE('',*,*,#14796,.T.);
#19769=ORIENTED_EDGE('',*,*,#14737,.F.);
#19770=ORIENTED_EDGE('',*,*,#14730,.F.);
#19771=ORIENTED_EDGE('',*,*,#14738,.F.);
#19772=ORIENTED_EDGE('',*,*,#14797,.T.);
#19773=ORIENTED_EDGE('',*,*,#14798,.F.);
#19774=ORIENTED_EDGE('',*,*,#14796,.F.);
#19775=ORIENTED_EDGE('',*,*,#14799,.F.);
#19776=ORIENTED_EDGE('',*,*,#14800,.F.);
#19777=ORIENTED_EDGE('',*,*,#14801,.F.);
#19778=ORIENTED_EDGE('',*,*,#14802,.F.);
#19779=ORIENTED_EDGE('',*,*,#14803,.F.);
#19780=ORIENTED_EDGE('',*,*,#14804,.F.);
#19781=ORIENTED_EDGE('',*,*,#14805,.T.);
#19782=ORIENTED_EDGE('',*,*,#14806,.T.);
#19783=ORIENTED_EDGE('',*,*,#14797,.F.);
#19784=ORIENTED_EDGE('',*,*,#14795,.F.);
#19785=ORIENTED_EDGE('',*,*,#14762,.F.);
#19786=ORIENTED_EDGE('',*,*,#14807,.T.);
#19787=ORIENTED_EDGE('',*,*,#14808,.T.);
#19788=ORIENTED_EDGE('',*,*,#14809,.F.);
#19789=ORIENTED_EDGE('',*,*,#14799,.T.);
#19790=ORIENTED_EDGE('',*,*,#14810,.F.);
#19791=ORIENTED_EDGE('',*,*,#14811,.F.);
#19792=ORIENTED_EDGE('',*,*,#14793,.F.);
#19793=ORIENTED_EDGE('',*,*,#14812,.T.);
#19794=ORIENTED_EDGE('',*,*,#14813,.T.);
#19795=ORIENTED_EDGE('',*,*,#14811,.T.);
#19796=ORIENTED_EDGE('',*,*,#14814,.T.);
#19797=ORIENTED_EDGE('',*,*,#14815,.T.);
#19798=ORIENTED_EDGE('',*,*,#14816,.T.);
#19799=ORIENTED_EDGE('',*,*,#14817,.T.);
#19800=ORIENTED_EDGE('',*,*,#14810,.T.);
#19801=ORIENTED_EDGE('',*,*,#14818,.T.);
#19802=ORIENTED_EDGE('',*,*,#14705,.F.);
#19803=ORIENTED_EDGE('',*,*,#14782,.F.);
#19804=ORIENTED_EDGE('',*,*,#14794,.F.);
#19805=ORIENTED_EDGE('',*,*,#14813,.F.);
#19806=ORIENTED_EDGE('',*,*,#14819,.F.);
#19807=ORIENTED_EDGE('',*,*,#14820,.F.);
#19808=ORIENTED_EDGE('',*,*,#14710,.F.);
#19809=ORIENTED_EDGE('',*,*,#14708,.F.);
#19810=ORIENTED_EDGE('',*,*,#14812,.F.);
#19811=ORIENTED_EDGE('',*,*,#14821,.T.);
#19812=ORIENTED_EDGE('',*,*,#14822,.T.);
#19813=ORIENTED_EDGE('',*,*,#14823,.F.);
#19814=ORIENTED_EDGE('',*,*,#14824,.T.);
#19815=ORIENTED_EDGE('',*,*,#14819,.T.);
#19816=ORIENTED_EDGE('',*,*,#14815,.F.);
#19817=ORIENTED_EDGE('',*,*,#14825,.T.);
#19818=ORIENTED_EDGE('',*,*,#14802,.T.);
#19819=ORIENTED_EDGE('',*,*,#14826,.T.);
#19820=ORIENTED_EDGE('',*,*,#14821,.F.);
#19821=ORIENTED_EDGE('',*,*,#14814,.F.);
#19822=ORIENTED_EDGE('',*,*,#14817,.F.);
#19823=ORIENTED_EDGE('',*,*,#14827,.T.);
#19824=ORIENTED_EDGE('',*,*,#14828,.T.);
#19825=ORIENTED_EDGE('',*,*,#14829,.T.);
#19826=ORIENTED_EDGE('',*,*,#14830,.F.);
#19827=ORIENTED_EDGE('',*,*,#14831,.F.);
#19828=ORIENTED_EDGE('',*,*,#14832,.F.);
#19829=ORIENTED_EDGE('',*,*,#14833,.F.);
#19830=ORIENTED_EDGE('',*,*,#14834,.F.);
#19831=ORIENTED_EDGE('',*,*,#14835,.T.);
#19832=ORIENTED_EDGE('',*,*,#14836,.T.);
#19833=ORIENTED_EDGE('',*,*,#14837,.F.);
#19834=ORIENTED_EDGE('',*,*,#14838,.F.);
#19835=ORIENTED_EDGE('',*,*,#14803,.T.);
#19836=ORIENTED_EDGE('',*,*,#14825,.F.);
#19837=ORIENTED_EDGE('',*,*,#14839,.T.);
#19838=ORIENTED_EDGE('',*,*,#14840,.T.);
#19839=ORIENTED_EDGE('',*,*,#14841,.T.);
#19840=ORIENTED_EDGE('',*,*,#14834,.T.);
#19841=ORIENTED_EDGE('',*,*,#14842,.T.);
#19842=ORIENTED_EDGE('',*,*,#14839,.F.);
#19843=ORIENTED_EDGE('',*,*,#14843,.F.);
#19844=ORIENTED_EDGE('',*,*,#14844,.T.);
#19845=ORIENTED_EDGE('',*,*,#14845,.T.);
#19846=ORIENTED_EDGE('',*,*,#14846,.T.);
#19847=ORIENTED_EDGE('',*,*,#14847,.T.);
#19848=ORIENTED_EDGE('',*,*,#14842,.F.);
#19849=ORIENTED_EDGE('',*,*,#14833,.T.);
#19850=ORIENTED_EDGE('',*,*,#14848,.F.);
#19851=ORIENTED_EDGE('',*,*,#14849,.F.);
#19852=ORIENTED_EDGE('',*,*,#14850,.T.);
#19853=ORIENTED_EDGE('',*,*,#14843,.T.);
#19854=ORIENTED_EDGE('',*,*,#14784,.T.);
#19855=ORIENTED_EDGE('',*,*,#14851,.T.);
#19856=ORIENTED_EDGE('',*,*,#14852,.T.);
#19857=ORIENTED_EDGE('',*,*,#14853,.T.);
#19858=ORIENTED_EDGE('',*,*,#14854,.T.);
#19859=ORIENTED_EDGE('',*,*,#14855,.T.);
#19860=ORIENTED_EDGE('',*,*,#14856,.T.);
#19861=ORIENTED_EDGE('',*,*,#14857,.T.);
#19862=ORIENTED_EDGE('',*,*,#14785,.T.);
#19863=ORIENTED_EDGE('',*,*,#14854,.F.);
#19864=ORIENTED_EDGE('',*,*,#14716,.F.);
#19865=ORIENTED_EDGE('',*,*,#14858,.F.);
#19866=ORIENTED_EDGE('',*,*,#14859,.T.);
#19867=ORIENTED_EDGE('',*,*,#14860,.F.);
#19868=ORIENTED_EDGE('',*,*,#14851,.F.);
#19869=ORIENTED_EDGE('',*,*,#14783,.T.);
#19870=ORIENTED_EDGE('',*,*,#14857,.F.);
#19871=ORIENTED_EDGE('',*,*,#14861,.F.);
#19872=ORIENTED_EDGE('',*,*,#14862,.T.);
#19873=ORIENTED_EDGE('',*,*,#14863,.F.);
#19874=ORIENTED_EDGE('',*,*,#14864,.F.);
#19875=ORIENTED_EDGE('',*,*,#14786,.T.);
#19876=ORIENTED_EDGE('',*,*,#14865,.T.);
#19877=ORIENTED_EDGE('',*,*,#14866,.T.);
#19878=ORIENTED_EDGE('',*,*,#14830,.T.);
#19879=ORIENTED_EDGE('',*,*,#14867,.T.);
#19880=ORIENTED_EDGE('',*,*,#14855,.F.);
#19881=ORIENTED_EDGE('',*,*,#14868,.F.);
#19882=ORIENTED_EDGE('',*,*,#14869,.F.);
#19883=ORIENTED_EDGE('',*,*,#14831,.T.);
#19884=ORIENTED_EDGE('',*,*,#14866,.F.);
#19885=ORIENTED_EDGE('',*,*,#14870,.T.);
#19886=ORIENTED_EDGE('',*,*,#14871,.T.);
#19887=ORIENTED_EDGE('',*,*,#14872,.F.);
#19888=ORIENTED_EDGE('',*,*,#14873,.F.);
#19889=ORIENTED_EDGE('',*,*,#14874,.F.);
#19890=ORIENTED_EDGE('',*,*,#14848,.T.);
#19891=ORIENTED_EDGE('',*,*,#14832,.T.);
#19892=ORIENTED_EDGE('',*,*,#14869,.T.);
#19893=ORIENTED_EDGE('',*,*,#14875,.T.);
#19894=ORIENTED_EDGE('',*,*,#14876,.T.);
#19895=ORIENTED_EDGE('',*,*,#14852,.F.);
#19896=ORIENTED_EDGE('',*,*,#14860,.T.);
#19897=ORIENTED_EDGE('',*,*,#14877,.T.);
#19898=ORIENTED_EDGE('',*,*,#14849,.T.);
#19899=ORIENTED_EDGE('',*,*,#14876,.F.);
#19900=ORIENTED_EDGE('',*,*,#14878,.T.);
#19901=ORIENTED_EDGE('',*,*,#14724,.T.);
#19902=ORIENTED_EDGE('',*,*,#14728,.T.);
#19903=ORIENTED_EDGE('',*,*,#14879,.T.);
#19904=ORIENTED_EDGE('',*,*,#14880,.T.);
#19905=ORIENTED_EDGE('',*,*,#14881,.T.);
#19906=ORIENTED_EDGE('',*,*,#14882,.T.);
#19907=ORIENTED_EDGE('',*,*,#14883,.T.);
#19908=ORIENTED_EDGE('',*,*,#14722,.T.);
#19909=ORIENTED_EDGE('',*,*,#14881,.F.);
#19910=ORIENTED_EDGE('',*,*,#14715,.F.);
#19911=ORIENTED_EDGE('',*,*,#14720,.T.);
#19912=ORIENTED_EDGE('',*,*,#14883,.F.);
#19913=ORIENTED_EDGE('',*,*,#14884,.T.);
#19914=ORIENTED_EDGE('',*,*,#14858,.T.);
#19915=ORIENTED_EDGE('',*,*,#14884,.F.);
#19916=ORIENTED_EDGE('',*,*,#14882,.F.);
#19917=ORIENTED_EDGE('',*,*,#14880,.F.);
#19918=ORIENTED_EDGE('',*,*,#14885,.F.);
#19919=ORIENTED_EDGE('',*,*,#14844,.F.);
#19920=ORIENTED_EDGE('',*,*,#14850,.F.);
#19921=ORIENTED_EDGE('',*,*,#14877,.F.);
#19922=ORIENTED_EDGE('',*,*,#14859,.F.);
#19923=ORIENTED_EDGE('',*,*,#14879,.F.);
#19924=ORIENTED_EDGE('',*,*,#14727,.F.);
#19925=ORIENTED_EDGE('',*,*,#14886,.T.);
#19926=ORIENTED_EDGE('',*,*,#14887,.F.);
#19927=ORIENTED_EDGE('',*,*,#14845,.F.);
#19928=ORIENTED_EDGE('',*,*,#14885,.T.);
#19929=ORIENTED_EDGE('',*,*,#14853,.F.);
#19930=ORIENTED_EDGE('',*,*,#14878,.F.);
#19931=ORIENTED_EDGE('',*,*,#14875,.F.);
#19932=ORIENTED_EDGE('',*,*,#14868,.T.);
#19933=ORIENTED_EDGE('',*,*,#14840,.F.);
#19934=ORIENTED_EDGE('',*,*,#14847,.F.);
#19935=ORIENTED_EDGE('',*,*,#14888,.F.);
#19936=ORIENTED_EDGE('',*,*,#14889,.T.);
#19937=ORIENTED_EDGE('',*,*,#14846,.F.);
#19938=ORIENTED_EDGE('',*,*,#14887,.T.);
#19939=ORIENTED_EDGE('',*,*,#14890,.T.);
#19940=ORIENTED_EDGE('',*,*,#14891,.T.);
#19941=ORIENTED_EDGE('',*,*,#14888,.T.);
#19942=ORIENTED_EDGE('',*,*,#14726,.F.);
#19943=ORIENTED_EDGE('',*,*,#14892,.F.);
#19944=ORIENTED_EDGE('',*,*,#14893,.F.);
#19945=ORIENTED_EDGE('',*,*,#14894,.F.);
#19946=ORIENTED_EDGE('',*,*,#14895,.F.);
#19947=ORIENTED_EDGE('',*,*,#14896,.F.);
#19948=ORIENTED_EDGE('',*,*,#14890,.F.);
#19949=ORIENTED_EDGE('',*,*,#14886,.F.);
#19950=ORIENTED_EDGE('',*,*,#14896,.T.);
#19951=ORIENTED_EDGE('',*,*,#14897,.T.);
#19952=ORIENTED_EDGE('',*,*,#14765,.T.);
#19953=ORIENTED_EDGE('',*,*,#14898,.T.);
#19954=ORIENTED_EDGE('',*,*,#14891,.F.);
#19955=ORIENTED_EDGE('',*,*,#14897,.F.);
#19956=ORIENTED_EDGE('',*,*,#14895,.T.);
#19957=ORIENTED_EDGE('',*,*,#14899,.F.);
#19958=ORIENTED_EDGE('',*,*,#14808,.F.);
#19959=ORIENTED_EDGE('',*,*,#14900,.T.);
#19960=ORIENTED_EDGE('',*,*,#14766,.T.);
#19961=ORIENTED_EDGE('',*,*,#14800,.T.);
#19962=ORIENTED_EDGE('',*,*,#14809,.T.);
#19963=ORIENTED_EDGE('',*,*,#14899,.T.);
#19964=ORIENTED_EDGE('',*,*,#14894,.T.);
#19965=ORIENTED_EDGE('',*,*,#14901,.T.);
#19966=ORIENTED_EDGE('',*,*,#14893,.T.);
#19967=ORIENTED_EDGE('',*,*,#14902,.T.);
#19968=ORIENTED_EDGE('',*,*,#14823,.T.);
#19969=ORIENTED_EDGE('',*,*,#14903,.T.);
#19970=ORIENTED_EDGE('',*,*,#14901,.F.);
#19971=ORIENTED_EDGE('',*,*,#14903,.F.);
#19972=ORIENTED_EDGE('',*,*,#14822,.F.);
#19973=ORIENTED_EDGE('',*,*,#14826,.F.);
#19974=ORIENTED_EDGE('',*,*,#14801,.T.);
#19975=ORIENTED_EDGE('',*,*,#14904,.T.);
#19976=ORIENTED_EDGE('',*,*,#14905,.T.);
#19977=ORIENTED_EDGE('',*,*,#14789,.F.);
#19978=ORIENTED_EDGE('',*,*,#14787,.T.);
#19979=ORIENTED_EDGE('',*,*,#14864,.T.);
#19980=ORIENTED_EDGE('',*,*,#14828,.F.);
#19981=ORIENTED_EDGE('',*,*,#14906,.T.);
#19982=ORIENTED_EDGE('',*,*,#14907,.T.);
#19983=ORIENTED_EDGE('',*,*,#14908,.T.);
#19984=ORIENTED_EDGE('',*,*,#14905,.F.);
#19985=ORIENTED_EDGE('',*,*,#14909,.F.);
#19986=ORIENTED_EDGE('',*,*,#14910,.F.);
#19987=ORIENTED_EDGE('',*,*,#14911,.F.);
#19988=ORIENTED_EDGE('',*,*,#14912,.F.);
#19989=ORIENTED_EDGE('',*,*,#14913,.T.);
#19990=ORIENTED_EDGE('',*,*,#14906,.F.);
#19991=ORIENTED_EDGE('',*,*,#14827,.F.);
#19992=ORIENTED_EDGE('',*,*,#14816,.F.);
#19993=ORIENTED_EDGE('',*,*,#14914,.F.);
#19994=ORIENTED_EDGE('',*,*,#14836,.F.);
#19995=ORIENTED_EDGE('',*,*,#14915,.T.);
#19996=ORIENTED_EDGE('',*,*,#14916,.T.);
#19997=ORIENTED_EDGE('',*,*,#14917,.T.);
#19998=ORIENTED_EDGE('',*,*,#14917,.F.);
#19999=ORIENTED_EDGE('',*,*,#14918,.F.);
#20000=ORIENTED_EDGE('',*,*,#14919,.F.);
#20001=ORIENTED_EDGE('',*,*,#14837,.T.);
#20002=ORIENTED_EDGE('',*,*,#14920,.F.);
#20003=ORIENTED_EDGE('',*,*,#14921,.F.);
#20004=ORIENTED_EDGE('',*,*,#14922,.T.);
#20005=ORIENTED_EDGE('',*,*,#14923,.T.);
#20006=ORIENTED_EDGE('',*,*,#14924,.T.);
#20007=ORIENTED_EDGE('',*,*,#14925,.T.);
#20008=ORIENTED_EDGE('',*,*,#14926,.T.);
#20009=ORIENTED_EDGE('',*,*,#14927,.F.);
#20010=ORIENTED_EDGE('',*,*,#14923,.F.);
#20011=ORIENTED_EDGE('',*,*,#14928,.F.);
#20012=ORIENTED_EDGE('',*,*,#14929,.F.);
#20013=ORIENTED_EDGE('',*,*,#14870,.F.);
#20014=ORIENTED_EDGE('',*,*,#14865,.F.);
#20015=ORIENTED_EDGE('',*,*,#14930,.F.);
#20016=ORIENTED_EDGE('',*,*,#14907,.F.);
#20017=ORIENTED_EDGE('',*,*,#14913,.F.);
#20018=ORIENTED_EDGE('',*,*,#14931,.F.);
#20019=ORIENTED_EDGE('',*,*,#14932,.F.);
#20020=ORIENTED_EDGE('',*,*,#14933,.F.);
#20021=ORIENTED_EDGE('',*,*,#14805,.F.);
#20022=ORIENTED_EDGE('',*,*,#14934,.F.);
#20023=ORIENTED_EDGE('',*,*,#14918,.T.);
#20024=ORIENTED_EDGE('',*,*,#14916,.F.);
#20025=ORIENTED_EDGE('',*,*,#14922,.F.);
#20026=ORIENTED_EDGE('',*,*,#14935,.F.);
#20027=ORIENTED_EDGE('',*,*,#14936,.T.);
#20028=ORIENTED_EDGE('',*,*,#14937,.T.);
#20029=ORIENTED_EDGE('',*,*,#14928,.T.);
#20030=ORIENTED_EDGE('',*,*,#14749,.F.);
#20031=ORIENTED_EDGE('',*,*,#14775,.T.);
#20032=ORIENTED_EDGE('',*,*,#14938,.T.);
#20033=ORIENTED_EDGE('',*,*,#14935,.T.);
#20034=ORIENTED_EDGE('',*,*,#14926,.F.);
#20035=ORIENTED_EDGE('',*,*,#14939,.T.);
#20036=ORIENTED_EDGE('',*,*,#14711,.F.);
#20037=ORIENTED_EDGE('',*,*,#14820,.T.);
#20038=ORIENTED_EDGE('',*,*,#14824,.F.);
#20039=ORIENTED_EDGE('',*,*,#14902,.F.);
#20040=ORIENTED_EDGE('',*,*,#14892,.T.);
#20041=ORIENTED_EDGE('',*,*,#14725,.F.);
#20042=ORIENTED_EDGE('',*,*,#14838,.T.);
#20043=ORIENTED_EDGE('',*,*,#14919,.T.);
#20044=ORIENTED_EDGE('',*,*,#14934,.T.);
#20045=ORIENTED_EDGE('',*,*,#14804,.T.);
#20046=ORIENTED_EDGE('',*,*,#14732,.F.);
#20047=ORIENTED_EDGE('',*,*,#14940,.T.);
#20048=ORIENTED_EDGE('',*,*,#14932,.T.);
#20049=ORIENTED_EDGE('',*,*,#14941,.T.);
#20050=ORIENTED_EDGE('',*,*,#14942,.T.);
#20051=ORIENTED_EDGE('',*,*,#14744,.T.);
#20052=ORIENTED_EDGE('',*,*,#14731,.F.);
#20053=ORIENTED_EDGE('',*,*,#14798,.T.);
#20054=ORIENTED_EDGE('',*,*,#14806,.F.);
#20055=ORIENTED_EDGE('',*,*,#14933,.T.);
#20056=ORIENTED_EDGE('',*,*,#14940,.F.);
#20057=ORIENTED_EDGE('',*,*,#14941,.F.);
#20058=ORIENTED_EDGE('',*,*,#14931,.T.);
#20059=ORIENTED_EDGE('',*,*,#14912,.T.);
#20060=ORIENTED_EDGE('',*,*,#14943,.T.);
#20061=ORIENTED_EDGE('',*,*,#14944,.F.);
#20062=ORIENTED_EDGE('',*,*,#14697,.T.);
#20063=ORIENTED_EDGE('',*,*,#14701,.T.);
#20064=ORIENTED_EDGE('',*,*,#14945,.T.);
#20065=ORIENTED_EDGE('',*,*,#14946,.T.);
#20066=ORIENTED_EDGE('',*,*,#14947,.T.);
#20067=ORIENTED_EDGE('',*,*,#14948,.T.);
#20068=ORIENTED_EDGE('',*,*,#14777,.T.);
#20069=ORIENTED_EDGE('',*,*,#14694,.T.);
#20070=ORIENTED_EDGE('',*,*,#14947,.F.);
#20071=ORIENTED_EDGE('',*,*,#14778,.F.);
#20072=ORIENTED_EDGE('',*,*,#14948,.F.);
#20073=ORIENTED_EDGE('',*,*,#14946,.F.);
#20074=ORIENTED_EDGE('',*,*,#14949,.F.);
#20075=ORIENTED_EDGE('',*,*,#14950,.F.);
#20076=ORIENTED_EDGE('',*,*,#14936,.F.);
#20077=ORIENTED_EDGE('',*,*,#14938,.F.);
#20078=ORIENTED_EDGE('',*,*,#14774,.F.);
#20079=ORIENTED_EDGE('',*,*,#14945,.F.);
#20080=ORIENTED_EDGE('',*,*,#14700,.F.);
#20081=ORIENTED_EDGE('',*,*,#14951,.T.);
#20082=ORIENTED_EDGE('',*,*,#14952,.F.);
#20083=ORIENTED_EDGE('',*,*,#14953,.F.);
#20084=ORIENTED_EDGE('',*,*,#14949,.T.);
#20085=ORIENTED_EDGE('',*,*,#14954,.F.);
#20086=ORIENTED_EDGE('',*,*,#14955,.F.);
#20087=ORIENTED_EDGE('',*,*,#14937,.F.);
#20088=ORIENTED_EDGE('',*,*,#14871,.F.);
#20089=ORIENTED_EDGE('',*,*,#14929,.T.);
#20090=ORIENTED_EDGE('',*,*,#14955,.T.);
#20091=ORIENTED_EDGE('',*,*,#14956,.T.);
#20092=ORIENTED_EDGE('',*,*,#14957,.T.);
#20093=ORIENTED_EDGE('',*,*,#14958,.T.);
#20094=ORIENTED_EDGE('',*,*,#14954,.T.);
#20095=ORIENTED_EDGE('',*,*,#14950,.T.);
#20096=ORIENTED_EDGE('',*,*,#14953,.T.);
#20097=ORIENTED_EDGE('',*,*,#14956,.F.);
#20098=ORIENTED_EDGE('',*,*,#14958,.F.);
#20099=ORIENTED_EDGE('',*,*,#14959,.F.);
#20100=ORIENTED_EDGE('',*,*,#14872,.T.);
#20101=ORIENTED_EDGE('',*,*,#14957,.F.);
#20102=ORIENTED_EDGE('',*,*,#14952,.T.);
#20103=ORIENTED_EDGE('',*,*,#14960,.T.);
#20104=ORIENTED_EDGE('',*,*,#14961,.T.);
#20105=ORIENTED_EDGE('',*,*,#14959,.T.);
#20106=ORIENTED_EDGE('',*,*,#14942,.F.);
#20107=ORIENTED_EDGE('',*,*,#14944,.T.);
#20108=ORIENTED_EDGE('',*,*,#14962,.T.);
#20109=ORIENTED_EDGE('',*,*,#14963,.T.);
#20110=ORIENTED_EDGE('',*,*,#14964,.T.);
#20111=ORIENTED_EDGE('',*,*,#14745,.T.);
#20112=ORIENTED_EDGE('',*,*,#14963,.F.);
#20113=ORIENTED_EDGE('',*,*,#14965,.T.);
#20114=ORIENTED_EDGE('',*,*,#14966,.F.);
#20115=ORIENTED_EDGE('',*,*,#14967,.T.);
#20116=ORIENTED_EDGE('',*,*,#14968,.T.);
#20117=ORIENTED_EDGE('',*,*,#14962,.F.);
#20118=ORIENTED_EDGE('',*,*,#14943,.F.);
#20119=ORIENTED_EDGE('',*,*,#14911,.T.);
#20120=ORIENTED_EDGE('',*,*,#14965,.F.);
#20121=ORIENTED_EDGE('',*,*,#14699,.F.);
#20122=ORIENTED_EDGE('',*,*,#14969,.F.);
#20123=ORIENTED_EDGE('',*,*,#14967,.F.);
#20124=ORIENTED_EDGE('',*,*,#14970,.F.);
#20125=ORIENTED_EDGE('',*,*,#14971,.F.);
#20126=ORIENTED_EDGE('',*,*,#14972,.F.);
#20127=ORIENTED_EDGE('',*,*,#14960,.F.);
#20128=ORIENTED_EDGE('',*,*,#14951,.F.);
#20129=ORIENTED_EDGE('',*,*,#14972,.T.);
#20130=ORIENTED_EDGE('',*,*,#14973,.T.);
#20131=ORIENTED_EDGE('',*,*,#14974,.T.);
#20132=ORIENTED_EDGE('',*,*,#14873,.T.);
#20133=ORIENTED_EDGE('',*,*,#14961,.F.);
#20134=ORIENTED_EDGE('',*,*,#14856,.F.);
#20135=ORIENTED_EDGE('',*,*,#14874,.T.);
#20136=ORIENTED_EDGE('',*,*,#14974,.F.);
#20137=ORIENTED_EDGE('',*,*,#14975,.F.);
#20138=ORIENTED_EDGE('',*,*,#14976,.T.);
#20139=ORIENTED_EDGE('',*,*,#14861,.T.);
#20140=ORIENTED_EDGE('',*,*,#14973,.F.);
#20141=ORIENTED_EDGE('',*,*,#14971,.T.);
#20142=ORIENTED_EDGE('',*,*,#14977,.F.);
#20143=ORIENTED_EDGE('',*,*,#14978,.F.);
#20144=ORIENTED_EDGE('',*,*,#14979,.T.);
#20145=ORIENTED_EDGE('',*,*,#14975,.T.);
#20146=ORIENTED_EDGE('',*,*,#14910,.T.);
#20147=ORIENTED_EDGE('',*,*,#14980,.T.);
#20148=ORIENTED_EDGE('',*,*,#14977,.T.);
#20149=ORIENTED_EDGE('',*,*,#14970,.T.);
#20150=ORIENTED_EDGE('',*,*,#14966,.T.);
#20151=ORIENTED_EDGE('',*,*,#14904,.F.);
#20152=ORIENTED_EDGE('',*,*,#14863,.T.);
#20153=ORIENTED_EDGE('',*,*,#14981,.T.);
#20154=ORIENTED_EDGE('',*,*,#14978,.T.);
#20155=ORIENTED_EDGE('',*,*,#14980,.F.);
#20156=ORIENTED_EDGE('',*,*,#14909,.T.);
#20157=ORIENTED_EDGE('',*,*,#14690,.F.);
#20158=ORIENTED_EDGE('',*,*,#14746,.T.);
#20159=ORIENTED_EDGE('',*,*,#14964,.F.);
#20160=ORIENTED_EDGE('',*,*,#14968,.F.);
#20161=ORIENTED_EDGE('',*,*,#14969,.T.);
#20162=ORIENTED_EDGE('',*,*,#14698,.F.);
#20163=ORIENTED_EDGE('',*,*,#14982,.T.);
#20164=ORIENTED_EDGE('',*,*,#14983,.T.);
#20165=ORIENTED_EDGE('',*,*,#14984,.T.);
#20166=ORIENTED_EDGE('',*,*,#14985,.T.);
#20167=ORIENTED_EDGE('',*,*,#14986,.T.);
#20168=ORIENTED_EDGE('',*,*,#14984,.F.);
#20169=ORIENTED_EDGE('',*,*,#14985,.F.);
#20170=ORIENTED_EDGE('',*,*,#14986,.F.);
#20171=ORIENTED_EDGE('',*,*,#14987,.T.);
#20172=ORIENTED_EDGE('',*,*,#14988,.F.);
#20173=ORIENTED_EDGE('',*,*,#14989,.F.);
#20174=ORIENTED_EDGE('',*,*,#14987,.F.);
#20175=ORIENTED_EDGE('',*,*,#14990,.F.);
#20176=ORIENTED_EDGE('',*,*,#14991,.T.);
#20177=ORIENTED_EDGE('',*,*,#14982,.F.);
#20178=ORIENTED_EDGE('',*,*,#14983,.F.);
#20179=ORIENTED_EDGE('',*,*,#14991,.F.);
#20180=ORIENTED_EDGE('',*,*,#14988,.T.);
#20181=ORIENTED_EDGE('',*,*,#14989,.T.);
#20182=ORIENTED_EDGE('',*,*,#14992,.T.);
#20183=ORIENTED_EDGE('',*,*,#14993,.T.);
#20184=ORIENTED_EDGE('',*,*,#14992,.F.);
#20185=ORIENTED_EDGE('',*,*,#14993,.F.);
#20186=ORIENTED_EDGE('',*,*,#14921,.T.);
#20187=ORIENTED_EDGE('',*,*,#14994,.T.);
#20188=ORIENTED_EDGE('',*,*,#14995,.T.);
#20189=ORIENTED_EDGE('',*,*,#14994,.F.);
#20190=ORIENTED_EDGE('',*,*,#14995,.F.);
#20191=ORIENTED_EDGE('',*,*,#14996,.T.);
#20192=ORIENTED_EDGE('',*,*,#14997,.F.);
#20193=ORIENTED_EDGE('',*,*,#14996,.F.);
#20194=ORIENTED_EDGE('',*,*,#14998,.T.);
#20195=ORIENTED_EDGE('',*,*,#14999,.T.);
#20196=ORIENTED_EDGE('',*,*,#14997,.T.);
#20197=ORIENTED_EDGE('',*,*,#14999,.F.);
#20198=ORIENTED_EDGE('',*,*,#14807,.F.);
#20199=ORIENTED_EDGE('',*,*,#14761,.F.);
#20200=ORIENTED_EDGE('',*,*,#14767,.F.);
#20201=ORIENTED_EDGE('',*,*,#14900,.F.);
#20202=ORIENTED_EDGE('',*,*,#15000,.F.);
#20203=ORIENTED_EDGE('',*,*,#14998,.F.);
#20204=ORIENTED_EDGE('',*,*,#14920,.T.);
#20205=ORIENTED_EDGE('',*,*,#15001,.T.);
#20206=ORIENTED_EDGE('',*,*,#15002,.T.);
#20207=ORIENTED_EDGE('',*,*,#15001,.F.);
#20208=ORIENTED_EDGE('',*,*,#15002,.F.);
#20209=ORIENTED_EDGE('',*,*,#15003,.T.);
#20210=ORIENTED_EDGE('',*,*,#15004,.F.);
#20211=ORIENTED_EDGE('',*,*,#15003,.F.);
#20212=ORIENTED_EDGE('',*,*,#15000,.T.);
#20213=ORIENTED_EDGE('',*,*,#15005,.T.);
#20214=ORIENTED_EDGE('',*,*,#15004,.T.);
#20215=ORIENTED_EDGE('',*,*,#15005,.F.);
#20216=ORIENTED_EDGE('',*,*,#15006,.F.);
#20217=ORIENTED_EDGE('',*,*,#15007,.T.);
#20218=ORIENTED_EDGE('',*,*,#14990,.T.);
#20219=ORIENTED_EDGE('',*,*,#15007,.F.);
#20220=ORIENTED_EDGE('',*,*,#14768,.F.);
#20221=ORIENTED_EDGE('',*,*,#14695,.T.);
#20222=ORIENTED_EDGE('',*,*,#14776,.F.);
#20223=ORIENTED_EDGE('',*,*,#14770,.F.);
#20224=ORIENTED_EDGE('',*,*,#14790,.F.);
#20225=ORIENTED_EDGE('',*,*,#14914,.T.);
#20226=ORIENTED_EDGE('',*,*,#14818,.F.);
#20227=ORIENTED_EDGE('',*,*,#14792,.F.);
#20228=ORIENTED_EDGE('',*,*,#14981,.F.);
#20229=ORIENTED_EDGE('',*,*,#14862,.F.);
#20230=ORIENTED_EDGE('',*,*,#14976,.F.);
#20231=ORIENTED_EDGE('',*,*,#14979,.F.);
#20232=ORIENTED_EDGE('',*,*,#15006,.T.);
#20233=ORIENTED_EDGE('',*,*,#14867,.F.);
#20234=ORIENTED_EDGE('',*,*,#14829,.F.);
#20235=ORIENTED_EDGE('',*,*,#14908,.F.);
#20236=ORIENTED_EDGE('',*,*,#14930,.T.);
#20237=ORIENTED_EDGE('',*,*,#14752,.F.);
#20238=ORIENTED_EDGE('',*,*,#15008,.F.);
#20239=ORIENTED_EDGE('',*,*,#14924,.F.);
#20240=ORIENTED_EDGE('',*,*,#14927,.T.);
#20241=ORIENTED_EDGE('',*,*,#14915,.F.);
#20242=ORIENTED_EDGE('',*,*,#14835,.F.);
#20243=ORIENTED_EDGE('',*,*,#14841,.F.);
#20244=ORIENTED_EDGE('',*,*,#14889,.F.);
#20245=ORIENTED_EDGE('',*,*,#14898,.F.);
#20246=ORIENTED_EDGE('',*,*,#14764,.F.);
#20247=ORIENTED_EDGE('',*,*,#14750,.F.);
#20248=ORIENTED_EDGE('',*,*,#14939,.F.);
#20249=ORIENTED_EDGE('',*,*,#14925,.F.);
#20250=ORIENTED_EDGE('',*,*,#15008,.T.);
#26172=PLANE('',#29046);
#26173=PLANE('',#29047);
#26174=PLANE('',#29048);
#26175=PLANE('',#29049);
#26176=PLANE('',#29050);
#26177=PLANE('',#29051);
#26178=PLANE('',#29052);
#26179=PLANE('',#29053);
#26180=PLANE('',#29054);
#26181=PLANE('',#29055);
#26182=PLANE('',#29056);
#26183=PLANE('',#29057);
#26184=PLANE('',#29058);
#26185=PLANE('',#29059);
#26186=PLANE('',#29060);
#26187=PLANE('',#29061);
#26188=PLANE('',#29062);
#26189=PLANE('',#29063);
#26190=PLANE('',#29064);
#26191=PLANE('',#29065);
#26192=PLANE('',#29066);
#26193=PLANE('',#29067);
#26194=PLANE('',#29068);
#26195=PLANE('',#29069);
#26196=PLANE('',#29070);
#26197=PLANE('',#29071);
#26198=PLANE('',#29072);
#26199=PLANE('',#29073);
#26200=PLANE('',#29074);
#26201=PLANE('',#29075);
#26202=PLANE('',#29076);
#26203=PLANE('',#29077);
#26204=PLANE('',#29078);
#26205=PLANE('',#29079);
#26206=PLANE('',#29080);
#26207=PLANE('',#29081);
#26208=PLANE('',#29082);
#26209=PLANE('',#29083);
#26210=PLANE('',#29084);
#26211=PLANE('',#29085);
#26212=PLANE('',#29086);
#26213=PLANE('',#29087);
#26214=PLANE('',#29088);
#26215=PLANE('',#29089);
#26216=PLANE('',#29090);
#26217=PLANE('',#29091);
#26218=PLANE('',#29092);
#26219=PLANE('',#29093);
#26220=PLANE('',#29094);
#26221=PLANE('',#29095);
#26222=PLANE('',#29096);
#26223=PLANE('',#29097);
#26224=PLANE('',#29098);
#26225=PLANE('',#29099);
#26226=PLANE('',#29100);
#26227=PLANE('',#29101);
#26228=PLANE('',#29102);
#26229=PLANE('',#29103);
#26230=PLANE('',#29104);
#26231=PLANE('',#29105);
#26232=PLANE('',#29106);
#26233=PLANE('',#29107);
#26234=PLANE('',#29108);
#26235=PLANE('',#29109);
#26236=PLANE('',#29110);
#26237=PLANE('',#29111);
#26238=PLANE('',#29112);
#26239=PLANE('',#29113);
#26240=PLANE('',#29114);
#26241=PLANE('',#29115);
#26242=PLANE('',#29116);
#26243=PLANE('',#29119);
#26244=PLANE('',#29120);
#26245=PLANE('',#29121);
#26246=PLANE('',#29122);
#26247=PLANE('',#29123);
#26248=PLANE('',#29124);
#26249=PLANE('',#29125);
#26250=PLANE('',#29126);
#26251=PLANE('',#29127);
#26252=PLANE('',#29128);
#26253=PLANE('',#29129);
#26254=PLANE('',#29130);
#26255=PLANE('',#29131);
#26256=PLANE('',#29132);
#26257=PLANE('',#29133);
#26258=PLANE('',#29134);
#26259=PLANE('',#29135);
#26260=PLANE('',#29136);
#26261=PLANE('',#29137);
#26262=PLANE('',#29138);
#26263=PLANE('',#29139);
#26264=PLANE('',#29140);
#26265=PLANE('',#29141);
#26266=PLANE('',#29142);
#26267=PLANE('',#29143);
#26268=PLANE('',#29144);
#26269=PLANE('',#29145);
#26270=PLANE('',#29146);
#26271=PLANE('',#29159);
#26272=PLANE('',#29166);
#26273=PLANE('',#29175);
#26274=PLANE('',#29176);
#26275=PLANE('',#29177);
#26276=PLANE('',#29178);
#26277=PLANE('',#29179);
#26278=PLANE('',#29180);
#27188=ADVANCED_FACE('',(#3280),#26172,.T.);
#27189=ADVANCED_FACE('',(#3281),#26173,.T.);
#27190=ADVANCED_FACE('',(#3282),#26174,.T.);
#27191=ADVANCED_FACE('',(#3283),#26175,.T.);
#27192=ADVANCED_FACE('',(#3284),#26176,.T.);
#27193=ADVANCED_FACE('',(#3285),#26177,.T.);
#27194=ADVANCED_FACE('',(#3286),#26178,.T.);
#27195=ADVANCED_FACE('',(#3287),#26179,.T.);
#27196=ADVANCED_FACE('',(#3288),#26180,.T.);
#27197=ADVANCED_FACE('',(#3289),#26181,.T.);
#27198=ADVANCED_FACE('',(#3290),#26182,.T.);
#27199=ADVANCED_FACE('',(#3291),#26183,.T.);
#27200=ADVANCED_FACE('',(#3292),#26184,.T.);
#27201=ADVANCED_FACE('',(#3293),#26185,.T.);
#27202=ADVANCED_FACE('',(#3294),#26186,.T.);
#27203=ADVANCED_FACE('',(#3295),#26187,.T.);
#27204=ADVANCED_FACE('',(#3296),#26188,.F.);
#27205=ADVANCED_FACE('',(#3297),#26189,.T.);
#27206=ADVANCED_FACE('',(#3298),#26190,.T.);
#27207=ADVANCED_FACE('',(#3299),#26191,.T.);
#27208=ADVANCED_FACE('',(#3300),#26192,.T.);
#27209=ADVANCED_FACE('',(#3301),#26193,.T.);
#27210=ADVANCED_FACE('',(#3302),#26194,.T.);
#27211=ADVANCED_FACE('',(#3303),#26195,.T.);
#27212=ADVANCED_FACE('',(#3304),#26196,.T.);
#27213=ADVANCED_FACE('',(#3305),#26197,.T.);
#27214=ADVANCED_FACE('',(#3306),#26198,.T.);
#27215=ADVANCED_FACE('',(#3307),#26199,.T.);
#27216=ADVANCED_FACE('',(#3308),#26200,.T.);
#27217=ADVANCED_FACE('',(#3309),#26201,.T.);
#27218=ADVANCED_FACE('',(#3310),#26202,.T.);
#27219=ADVANCED_FACE('',(#3311),#26203,.T.);
#27220=ADVANCED_FACE('',(#3312),#26204,.T.);
#27221=ADVANCED_FACE('',(#3313),#26205,.T.);
#27222=ADVANCED_FACE('',(#3314),#26206,.T.);
#27223=ADVANCED_FACE('',(#3315),#26207,.T.);
#27224=ADVANCED_FACE('',(#3316),#26208,.T.);
#27225=ADVANCED_FACE('',(#3317),#26209,.F.);
#27226=ADVANCED_FACE('',(#3318),#26210,.T.);
#27227=ADVANCED_FACE('',(#3319),#26211,.T.);
#27228=ADVANCED_FACE('',(#3320),#26212,.T.);
#27229=ADVANCED_FACE('',(#3321),#26213,.T.);
#27230=ADVANCED_FACE('',(#3322),#26214,.T.);
#27231=ADVANCED_FACE('',(#3323),#26215,.T.);
#27232=ADVANCED_FACE('',(#3324),#26216,.T.);
#27233=ADVANCED_FACE('',(#3325),#26217,.T.);
#27234=ADVANCED_FACE('',(#3326),#26218,.T.);
#27235=ADVANCED_FACE('',(#3327),#26219,.T.);
#27236=ADVANCED_FACE('',(#3328),#26220,.T.);
#27237=ADVANCED_FACE('',(#3329),#26221,.T.);
#27238=ADVANCED_FACE('',(#3330),#26222,.T.);
#27239=ADVANCED_FACE('',(#3331),#26223,.T.);
#27240=ADVANCED_FACE('',(#3332),#26224,.T.);
#27241=ADVANCED_FACE('',(#3333),#26225,.T.);
#27242=ADVANCED_FACE('',(#3334),#26226,.T.);
#27243=ADVANCED_FACE('',(#3335),#26227,.T.);
#27244=ADVANCED_FACE('',(#3336),#26228,.T.);
#27245=ADVANCED_FACE('',(#3337),#26229,.T.);
#27246=ADVANCED_FACE('',(#3338),#26230,.T.);
#27247=ADVANCED_FACE('',(#3339),#26231,.T.);
#27248=ADVANCED_FACE('',(#3340),#26232,.T.);
#27249=ADVANCED_FACE('',(#3341),#26233,.T.);
#27250=ADVANCED_FACE('',(#3342),#26234,.T.);
#27251=ADVANCED_FACE('',(#3343),#26235,.T.);
#27252=ADVANCED_FACE('',(#3344),#26236,.T.);
#27253=ADVANCED_FACE('',(#3345),#26237,.T.);
#27254=ADVANCED_FACE('',(#3346),#26238,.T.);
#27255=ADVANCED_FACE('',(#3347),#26239,.T.);
#27256=ADVANCED_FACE('',(#3348),#26240,.T.);
#27257=ADVANCED_FACE('',(#3349),#26241,.T.);
#27258=ADVANCED_FACE('',(#3350,#1905,#1906),#26242,.F.);
#27259=ADVANCED_FACE('',(#3351),#26243,.T.);
#27260=ADVANCED_FACE('',(#3352),#26244,.T.);
#27261=ADVANCED_FACE('',(#3353),#26245,.T.);
#27262=ADVANCED_FACE('',(#3354),#26246,.T.);
#27263=ADVANCED_FACE('',(#3355),#26247,.T.);
#27264=ADVANCED_FACE('',(#3356),#26248,.T.);
#27265=ADVANCED_FACE('',(#3357),#26249,.T.);
#27266=ADVANCED_FACE('',(#3358),#26250,.T.);
#27267=ADVANCED_FACE('',(#3359),#26251,.T.);
#27268=ADVANCED_FACE('',(#3360),#26252,.T.);
#27269=ADVANCED_FACE('',(#3361),#26253,.T.);
#27270=ADVANCED_FACE('',(#3362),#26254,.T.);
#27271=ADVANCED_FACE('',(#3363),#26255,.T.);
#27272=ADVANCED_FACE('',(#3364),#26256,.T.);
#27273=ADVANCED_FACE('',(#3365),#26257,.T.);
#27274=ADVANCED_FACE('',(#3366),#26258,.T.);
#27275=ADVANCED_FACE('',(#3367),#26259,.T.);
#27276=ADVANCED_FACE('',(#3368),#26260,.T.);
#27277=ADVANCED_FACE('',(#3369),#26261,.T.);
#27278=ADVANCED_FACE('',(#3370),#26262,.T.);
#27279=ADVANCED_FACE('',(#3371),#26263,.T.);
#27280=ADVANCED_FACE('',(#3372),#26264,.T.);
#27281=ADVANCED_FACE('',(#3373),#26265,.T.);
#27282=ADVANCED_FACE('',(#3374),#26266,.T.);
#27283=ADVANCED_FACE('',(#3375),#26267,.T.);
#27284=ADVANCED_FACE('',(#3376),#26268,.T.);
#27285=ADVANCED_FACE('',(#3377),#26269,.T.);
#27286=ADVANCED_FACE('',(#3378),#26270,.T.);
#27287=ADVANCED_FACE('',(#3379),#2799,.T.);
#27288=ADVANCED_FACE('',(#3380),#2800,.T.);
#27289=ADVANCED_FACE('',(#3381),#1566,.T.);
#27290=ADVANCED_FACE('',(#3382),#2801,.T.);
#27291=ADVANCED_FACE('',(#3383),#26271,.T.);
#27292=ADVANCED_FACE('',(#3384),#2802,.F.);
#27293=ADVANCED_FACE('',(#3385),#1567,.F.);
#27294=ADVANCED_FACE('',(#3386),#2803,.F.);
#27295=ADVANCED_FACE('',(#3387,#1907,#1908),#26272,.T.);
#27296=ADVANCED_FACE('',(#3388),#2804,.F.);
#27297=ADVANCED_FACE('',(#3389),#1568,.F.);
#27298=ADVANCED_FACE('',(#3390),#2805,.F.);
#27299=ADVANCED_FACE('',(#3391),#2806,.T.);
#27300=ADVANCED_FACE('',(#3392),#26273,.T.);
#27301=ADVANCED_FACE('',(#3393),#26274,.T.);
#27302=ADVANCED_FACE('',(#3394,#1909),#26275,.F.);
#27303=ADVANCED_FACE('',(#3395),#26276,.T.);
#27304=ADVANCED_FACE('',(#3396),#26277,.T.);
#27305=ADVANCED_FACE('',(#3397),#26278,.T.);
#28460=CLOSED_SHELL('',(#27188,#27189,#27190,#27191,#27192,#27193,#27194,
#27195,#27196,#27197,#27198,#27199,#27200,#27201,#27202,#27203,#27204,#27205,
#27206,#27207,#27208,#27209,#27210,#27211,#27212,#27213,#27214,#27215,#27216,
#27217,#27218,#27219,#27220,#27221,#27222,#27223,#27224,#27225,#27226,#27227,
#27228,#27229,#27230,#27231,#27232,#27233,#27234,#27235,#27236,#27237,#27238,
#27239,#27240,#27241,#27242,#27243,#27244,#27245,#27246,#27247,#27248,#27249,
#27250,#27251,#27252,#27253,#27254,#27255,#27256,#27257,#27258,#27259,#27260,
#27261,#27262,#27263,#27264,#27265,#27266,#27267,#27268,#27269,#27270,#27271,
#27272,#27273,#27274,#27275,#27276,#27277,#27278,#27279,#27280,#27281,#27282,
#27283,#27284,#27285,#27286,#27287,#27288,#27289,#27290,#27291,#27292,#27293,
#27294,#27295,#27296,#27297,#27298,#27299,#27300,#27301,#27302,#27303,#27304,
#27305));
#29045=AXIS2_PLACEMENT_3D('',#42153,#32025,#32026);
#29046=AXIS2_PLACEMENT_3D('',#42154,#32027,#32028);
#29047=AXIS2_PLACEMENT_3D('',#42163,#32033,#32034);
#29048=AXIS2_PLACEMENT_3D('',#42171,#32039,#32040);
#29049=AXIS2_PLACEMENT_3D('',#42177,#32044,#32045);
#29050=AXIS2_PLACEMENT_3D('',#42181,#32048,#32049);
#29051=AXIS2_PLACEMENT_3D('',#42189,#32054,#32055);
#29052=AXIS2_PLACEMENT_3D('',#42200,#32061,#32062);
#29053=AXIS2_PLACEMENT_3D('',#42206,#32066,#32067);
#29054=AXIS2_PLACEMENT_3D('',#42214,#32072,#32073);
#29055=AXIS2_PLACEMENT_3D('',#42224,#32079,#32080);
#29056=AXIS2_PLACEMENT_3D('',#42228,#32083,#32084);
#29057=AXIS2_PLACEMENT_3D('',#42232,#32087,#32088);
#29058=AXIS2_PLACEMENT_3D('',#42236,#32091,#32092);
#29059=AXIS2_PLACEMENT_3D('',#42244,#32097,#32098);
#29060=AXIS2_PLACEMENT_3D('',#42257,#32105,#32106);
#29061=AXIS2_PLACEMENT_3D('',#42265,#32111,#32112);
#29062=AXIS2_PLACEMENT_3D('',#42273,#32117,#32118);
#29063=AXIS2_PLACEMENT_3D('',#42280,#32123,#32124);
#29064=AXIS2_PLACEMENT_3D('',#42291,#32130,#32131);
#29065=AXIS2_PLACEMENT_3D('',#42299,#32136,#32137);
#29066=AXIS2_PLACEMENT_3D('',#42306,#32142,#32143);
#29067=AXIS2_PLACEMENT_3D('',#42314,#32148,#32149);
#29068=AXIS2_PLACEMENT_3D('',#42322,#32154,#32155);
#29069=AXIS2_PLACEMENT_3D('',#42326,#32158,#32159);
#29070=AXIS2_PLACEMENT_3D('',#42332,#32163,#32164);
#29071=AXIS2_PLACEMENT_3D('',#42338,#32168,#32169);
#29072=AXIS2_PLACEMENT_3D('',#42343,#32173,#32174);
#29073=AXIS2_PLACEMENT_3D('',#42351,#32179,#32180);
#29074=AXIS2_PLACEMENT_3D('',#42363,#32187,#32188);
#29075=AXIS2_PLACEMENT_3D('',#42369,#32192,#32193);
#29076=AXIS2_PLACEMENT_3D('',#42375,#32197,#32198);
#29077=AXIS2_PLACEMENT_3D('',#42379,#32201,#32202);
#29078=AXIS2_PLACEMENT_3D('',#42383,#32205,#32206);
#29079=AXIS2_PLACEMENT_3D('',#42399,#32215,#32216);
#29080=AXIS2_PLACEMENT_3D('',#42405,#32220,#32221);
#29081=AXIS2_PLACEMENT_3D('',#42409,#32224,#32225);
#29082=AXIS2_PLACEMENT_3D('',#42417,#32230,#32231);
#29083=AXIS2_PLACEMENT_3D('',#42423,#32235,#32236);
#29084=AXIS2_PLACEMENT_3D('',#42427,#32239,#32240);
#29085=AXIS2_PLACEMENT_3D('',#42435,#32245,#32246);
#29086=AXIS2_PLACEMENT_3D('',#42438,#32249,#32250);
#29087=AXIS2_PLACEMENT_3D('',#42462,#32263,#32264);
#29088=AXIS2_PLACEMENT_3D('',#42470,#32269,#32270);
#29089=AXIS2_PLACEMENT_3D('',#42480,#32276,#32277);
#29090=AXIS2_PLACEMENT_3D('',#42486,#32281,#32282);
#29091=AXIS2_PLACEMENT_3D('',#42494,#32287,#32288);
#29092=AXIS2_PLACEMENT_3D('',#42500,#32292,#32293);
#29093=AXIS2_PLACEMENT_3D('',#42506,#32297,#32298);
#29094=AXIS2_PLACEMENT_3D('',#42514,#32303,#32304);
#29095=AXIS2_PLACEMENT_3D('',#42520,#32308,#32309);
#29096=AXIS2_PLACEMENT_3D('',#42533,#32317,#32318);
#29097=AXIS2_PLACEMENT_3D('',#42537,#32321,#32322);
#29098=AXIS2_PLACEMENT_3D('',#42540,#32325,#32326);
#29099=AXIS2_PLACEMENT_3D('',#42546,#32330,#32331);
#29100=AXIS2_PLACEMENT_3D('',#42550,#32334,#32335);
#29101=AXIS2_PLACEMENT_3D('',#42552,#32337,#32338);
#29102=AXIS2_PLACEMENT_3D('',#42554,#32340,#32341);
#29103=AXIS2_PLACEMENT_3D('',#42558,#32344,#32345);
#29104=AXIS2_PLACEMENT_3D('',#42559,#32346,#32347);
#29105=AXIS2_PLACEMENT_3D('',#42563,#32350,#32351);
#29106=AXIS2_PLACEMENT_3D('',#42567,#32354,#32355);
#29107=AXIS2_PLACEMENT_3D('',#42577,#32361,#32362);
#29108=AXIS2_PLACEMENT_3D('',#42580,#32365,#32366);
#29109=AXIS2_PLACEMENT_3D('',#42583,#32369,#32370);
#29110=AXIS2_PLACEMENT_3D('',#42585,#32372,#32373);
#29111=AXIS2_PLACEMENT_3D('',#42588,#32376,#32377);
#29112=AXIS2_PLACEMENT_3D('',#42589,#32378,#32379);
#29113=AXIS2_PLACEMENT_3D('',#42593,#32382,#32383);
#29114=AXIS2_PLACEMENT_3D('',#42599,#32387,#32388);
#29115=AXIS2_PLACEMENT_3D('',#42610,#32395,#32396);
#29116=AXIS2_PLACEMENT_3D('',#42616,#32400,#32401);
#29117=AXIS2_PLACEMENT_3D('',#42621,#32404,#32405);
#29118=AXIS2_PLACEMENT_3D('',#42623,#32406,#32407);
#29119=AXIS2_PLACEMENT_3D('',#42624,#32408,#32409);
#29120=AXIS2_PLACEMENT_3D('',#42635,#32415,#32416);
#29121=AXIS2_PLACEMENT_3D('',#42647,#32425,#32426);
#29122=AXIS2_PLACEMENT_3D('',#42653,#32430,#32431);
#29123=AXIS2_PLACEMENT_3D('',#42656,#32434,#32435);
#29124=AXIS2_PLACEMENT_3D('',#42657,#32436,#32437);
#29125=AXIS2_PLACEMENT_3D('',#42658,#32438,#32439);
#29126=AXIS2_PLACEMENT_3D('',#42663,#32443,#32444);
#29127=AXIS2_PLACEMENT_3D('',#42664,#32445,#32446);
#29128=AXIS2_PLACEMENT_3D('',#42668,#32449,#32450);
#29129=AXIS2_PLACEMENT_3D('',#42674,#32454,#32455);
#29130=AXIS2_PLACEMENT_3D('',#42676,#32457,#32458);
#29131=AXIS2_PLACEMENT_3D('',#42680,#32461,#32462);
#29132=AXIS2_PLACEMENT_3D('',#42686,#32466,#32467);
#29133=AXIS2_PLACEMENT_3D('',#42690,#32470,#32471);
#29134=AXIS2_PLACEMENT_3D('',#42692,#32473,#32474);
#29135=AXIS2_PLACEMENT_3D('',#42696,#32477,#32478);
#29136=AXIS2_PLACEMENT_3D('',#42698,#32480,#32481);
#29137=AXIS2_PLACEMENT_3D('',#42702,#32484,#32485);
#29138=AXIS2_PLACEMENT_3D('',#42708,#32489,#32490);
#29139=AXIS2_PLACEMENT_3D('',#42715,#32495,#32496);
#29140=AXIS2_PLACEMENT_3D('',#42716,#32497,#32498);
#29141=AXIS2_PLACEMENT_3D('',#42723,#32503,#32504);
#29142=AXIS2_PLACEMENT_3D('',#42727,#32507,#32508);
#29143=AXIS2_PLACEMENT_3D('',#42731,#32511,#32512);
#29144=AXIS2_PLACEMENT_3D('',#42737,#32516,#32517);
#29145=AXIS2_PLACEMENT_3D('',#42739,#32519,#32520);
#29146=AXIS2_PLACEMENT_3D('',#42741,#32522,#32523);
#29147=AXIS2_PLACEMENT_3D('',#42742,#32524,#32525);
#29148=AXIS2_PLACEMENT_3D('',#42745,#32526,#32527);
#29149=AXIS2_PLACEMENT_3D('',#42746,#32528,#32529);
#29150=AXIS2_PLACEMENT_3D('',#42750,#32531,#32532);
#29151=AXIS2_PLACEMENT_3D('',#42751,#32533,#32534);
#29152=AXIS2_PLACEMENT_3D('',#42752,#32535,#32536);
#29153=AXIS2_PLACEMENT_3D('',#42756,#32538,#32539);
#29154=AXIS2_PLACEMENT_3D('',#42757,#32540,#32541);
#29155=AXIS2_PLACEMENT_3D('',#42758,#32542,#32543);
#29156=AXIS2_PLACEMENT_3D('',#42760,#32544,#32545);
#29157=AXIS2_PLACEMENT_3D('',#42762,#32547,#32548);
#29158=AXIS2_PLACEMENT_3D('',#42765,#32550,#32551);
#29159=AXIS2_PLACEMENT_3D('',#42766,#32552,#32553);
#29160=AXIS2_PLACEMENT_3D('',#42767,#32554,#32555);
#29161=AXIS2_PLACEMENT_3D('',#42770,#32557,#32558);
#29162=AXIS2_PLACEMENT_3D('',#42771,#32559,#32560);
#29163=AXIS2_PLACEMENT_3D('',#42774,#32562,#32563);
#29164=AXIS2_PLACEMENT_3D('',#42775,#32564,#32565);
#29165=AXIS2_PLACEMENT_3D('',#42777,#32566,#32567);
#29166=AXIS2_PLACEMENT_3D('',#42779,#32569,#32570);
#29167=AXIS2_PLACEMENT_3D('',#42781,#32571,#32572);
#29168=AXIS2_PLACEMENT_3D('',#42782,#32573,#32574);
#29169=AXIS2_PLACEMENT_3D('',#42785,#32576,#32577);
#29170=AXIS2_PLACEMENT_3D('',#42786,#32578,#32579);
#29171=AXIS2_PLACEMENT_3D('',#42789,#32581,#32582);
#29172=AXIS2_PLACEMENT_3D('',#42790,#32583,#32584);
#29173=AXIS2_PLACEMENT_3D('',#42792,#32586,#32587);
#29174=AXIS2_PLACEMENT_3D('',#42794,#32588,#32589);
#29175=AXIS2_PLACEMENT_3D('',#42796,#32591,#32592);
#29176=AXIS2_PLACEMENT_3D('',#42797,#32593,#32594);
#29177=AXIS2_PLACEMENT_3D('',#42798,#32595,#32596);
#29178=AXIS2_PLACEMENT_3D('',#42799,#32597,#32598);
#29179=AXIS2_PLACEMENT_3D('',#42800,#32599,#32600);
#29180=AXIS2_PLACEMENT_3D('',#42802,#32602,#32603);
#32025=DIRECTION('axis',(0.,0.,1.));
#32026=DIRECTION('refdir',(1.,0.,0.));
#32027=DIRECTION('center_axis',(-0.707106781186544,-0.707106781186551,0.));
#32028=DIRECTION('ref_axis',(0.,0.,1.));
#32029=DIRECTION('',(0.,0.,1.));
#32030=DIRECTION('',(0.577350269189641,-0.577350269189636,-0.5773502691896));
#32031=DIRECTION('',(0.,0.,-1.));
#32032=DIRECTION('',(0.577350269189641,-0.577350269189636,0.5773502691896));
#32033=DIRECTION('center_axis',(-0.707106781186522,0.,0.707106781186573));
#32034=DIRECTION('ref_axis',(0.707106781186573,0.,0.707106781186522));
#32035=DIRECTION('',(0.,-1.,0.));
#32036=DIRECTION('',(0.577350269189643,-0.577350269189633,0.577350269189602));
#32037=DIRECTION('',(0.577350269189643,0.577350269189633,0.577350269189602));
#32038=DIRECTION('',(0.,1.,0.));
#32039=DIRECTION('center_axis',(0.,-1.,0.));
#32040=DIRECTION('ref_axis',(0.,0.,-1.));
#32041=DIRECTION('',(1.,0.,0.));
#32042=DIRECTION('',(0.,0.,-1.));
#32043=DIRECTION('',(1.,0.,0.));
#32044=DIRECTION('center_axis',(0.,0.,1.));
#32045=DIRECTION('ref_axis',(0.,-1.,0.));
#32046=DIRECTION('',(-1.,0.,0.));
#32047=DIRECTION('',(0.,-1.,0.));
#32048=DIRECTION('center_axis',(0.,-0.707106781186529,0.707106781186566));
#32049=DIRECTION('ref_axis',(1.,0.,0.));
#32050=DIRECTION('',(0.577350269189643,-0.577350269189633,-0.577350269189602));
#32051=DIRECTION('',(1.,0.,0.));
#32052=DIRECTION('',(0.577350269189616,0.577350269189646,0.577350269189616));
#32053=DIRECTION('',(0.577350269189616,-0.577350269189646,-0.577350269189616));
#32054=DIRECTION('center_axis',(-0.707106781186548,0.,0.707106781186548));
#32055=DIRECTION('ref_axis',(0.707106781186548,0.,0.707106781186548));
#32056=DIRECTION('',(0.,1.,0.));
#32057=DIRECTION('',(-0.577350269189616,0.577350269189646,-0.577350269189616));
#32058=DIRECTION('',(-0.577350269189616,-0.577350269189646,-0.577350269189616));
#32059=DIRECTION('',(0.,-1.,0.));
#32060=DIRECTION('',(0.577350269189616,0.577350269189646,0.577350269189616));
#32061=DIRECTION('center_axis',(-0.707106781186566,0.707106781186529,0.));
#32062=DIRECTION('ref_axis',(0.,0.,1.));
#32063=DIRECTION('',(0.,0.,-1.));
#32064=DIRECTION('',(0.,0.,1.));
#32065=DIRECTION('',(0.577350269189616,0.577350269189646,-0.577350269189616));
#32066=DIRECTION('center_axis',(-0.707106781186548,0.,-0.707106781186548));
#32067=DIRECTION('ref_axis',(-0.707106781186548,0.,0.707106781186548));
#32068=DIRECTION('',(0.,1.,0.));
#32069=DIRECTION('',(0.577350269189616,0.577350269189646,-0.577350269189616));
#32070=DIRECTION('',(0.577350269189616,-0.577350269189646,-0.577350269189616));
#32071=DIRECTION('',(0.,-1.,0.));
#32072=DIRECTION('center_axis',(0.,0.707106781186529,0.707106781186566));
#32073=DIRECTION('ref_axis',(1.,0.,0.));
#32074=DIRECTION('',(1.,0.,0.));
#32075=DIRECTION('',(0.577350269189616,0.577350269189646,-0.577350269189616));
#32076=DIRECTION('',(-0.577350269189616,0.577350269189646,-0.577350269189616));
#32077=DIRECTION('',(-1.,0.,0.));
#32078=DIRECTION('',(-0.577350269189616,-0.577350269189646,0.577350269189616));
#32079=DIRECTION('center_axis',(0.,0.,1.));
#32080=DIRECTION('ref_axis',(0.,-1.,0.));
#32081=DIRECTION('',(1.,0.,0.));
#32082=DIRECTION('',(0.,-1.,0.));
#32083=DIRECTION('center_axis',(0.,1.,0.));
#32084=DIRECTION('ref_axis',(0.,0.,1.));
#32085=DIRECTION('',(1.,0.,0.));
#32086=DIRECTION('',(0.,0.,1.));
#32087=DIRECTION('center_axis',(0.,0.,-1.));
#32088=DIRECTION('ref_axis',(0.,1.,0.));
#32089=DIRECTION('',(-1.,0.,0.));
#32090=DIRECTION('',(0.,1.,0.));
#32091=DIRECTION('center_axis',(0.,0.707106781186529,-0.707106781186566));
#32092=DIRECTION('ref_axis',(-1.,0.,0.));
#32093=DIRECTION('',(0.577350269189616,0.577350269189646,0.577350269189616));
#32094=DIRECTION('',(1.,0.,0.));
#32095=DIRECTION('',(0.577350269189616,-0.577350269189646,-0.577350269189616));
#32096=DIRECTION('',(0.577350269189616,0.577350269189646,0.577350269189616));
#32097=DIRECTION('center_axis',(-0.707106781186522,0.,0.707106781186573));
#32098=DIRECTION('ref_axis',(0.707106781186573,0.,0.707106781186522));
#32099=DIRECTION('',(0.577350269189643,0.577350269189633,0.577350269189602));
#32100=DIRECTION('',(0.,1.,0.));
#32101=DIRECTION('',(-0.577350269189643,0.577350269189633,-0.577350269189602));
#32102=DIRECTION('',(-0.577350269189643,-0.577350269189633,-0.577350269189602));
#32103=DIRECTION('',(0.,-1.,0.));
#32104=DIRECTION('',(0.577350269189643,-0.577350269189633,0.577350269189602));
#32105=DIRECTION('center_axis',(0.,-0.707106781186529,0.707106781186566));
#32106=DIRECTION('ref_axis',(1.,0.,0.));
#32107=DIRECTION('',(0.577350269189643,-0.577350269189633,-0.577350269189602));
#32108=DIRECTION('',(1.,0.,0.));
#32109=DIRECTION('',(-0.577350269189616,0.577350269189646,0.577350269189616));
#32110=DIRECTION('',(-1.,0.,0.));
#32111=DIRECTION('center_axis',(-0.707106781186541,-0.707106781186554,0.));
#32112=DIRECTION('ref_axis',(0.,0.,1.));
#32113=DIRECTION('',(0.,0.,-1.));
#32114=DIRECTION('',(-0.577350269189643,0.577350269189633,0.577350269189602));
#32115=DIRECTION('',(-0.577350269189643,0.577350269189633,-0.577350269189602));
#32116=DIRECTION('',(0.,0.,1.));
#32117=DIRECTION('center_axis',(1.,0.,0.));
#32118=DIRECTION('ref_axis',(0.,0.,-1.));
#32119=DIRECTION('',(0.,1.,0.));
#32120=DIRECTION('',(0.,0.,1.));
#32121=DIRECTION('',(0.,1.,0.));
#32122=DIRECTION('',(0.,0.,-1.));
#32123=DIRECTION('center_axis',(0.,-0.707106781186529,0.707106781186566));
#32124=DIRECTION('ref_axis',(1.,0.,0.));
#32125=DIRECTION('',(1.,0.,0.));
#32126=DIRECTION('',(0.577350269189616,0.577350269189646,0.577350269189616));
#32127=DIRECTION('',(-0.577350269189616,0.577350269189646,0.577350269189616));
#32128=DIRECTION('',(-1.,0.,0.));
#32129=DIRECTION('',(-0.577350269189616,-0.577350269189646,-0.577350269189616));
#32130=DIRECTION('center_axis',(0.707106781186554,-0.707106781186541,0.));
#32131=DIRECTION('ref_axis',(0.,0.,-1.));
#32132=DIRECTION('',(0.,0.,1.));
#32133=DIRECTION('',(-0.577350269189613,-0.577350269189624,0.577350269189641));
#32134=DIRECTION('',(-0.577350269189612,-0.577350269189622,-0.577350269189643));
#32135=DIRECTION('',(0.,0.,-1.));
#32136=DIRECTION('center_axis',(0.,-1.,0.));
#32137=DIRECTION('ref_axis',(0.,0.,-1.));
#32138=DIRECTION('',(1.,0.,0.));
#32139=DIRECTION('',(0.,0.,1.));
#32140=DIRECTION('',(-1.,0.,0.));
#32141=DIRECTION('',(0.,0.,-1.));
#32142=DIRECTION('center_axis',(0.,-0.70710678118656,0.707106781186535));
#32143=DIRECTION('ref_axis',(1.,0.,0.));
#32144=DIRECTION('',(0.577350269189605,-0.577350269189626,-0.577350269189646));
#32145=DIRECTION('',(-1.,0.,0.));
#32146=DIRECTION('',(-0.577350269189614,-0.577350269189621,-0.577350269189642));
#32147=DIRECTION('',(-0.577350269189612,0.577350269189622,0.577350269189643));
#32148=DIRECTION('center_axis',(0.707106781186564,0.,0.707106781186531));
#32149=DIRECTION('ref_axis',(0.707106781186531,0.,-0.707106781186564));
#32150=DIRECTION('',(0.,1.,0.));
#32151=DIRECTION('',(0.577350269189613,-0.577350269189624,-0.577350269189641));
#32152=DIRECTION('',(0.577350269189614,0.577350269189621,-0.577350269189642));
#32153=DIRECTION('',(0.,-1.,0.));
#32154=DIRECTION('center_axis',(-0.707106781186522,0.,-0.707106781186573));
#32155=DIRECTION('ref_axis',(-0.707106781186573,0.,0.707106781186522));
#32156=DIRECTION('',(0.,-1.,0.));
#32157=DIRECTION('',(-0.577350269189643,-0.577350269189633,0.577350269189602));
#32158=DIRECTION('center_axis',(0.,-0.707106781186529,-0.707106781186566));
#32159=DIRECTION('ref_axis',(-1.,0.,0.));
#32160=DIRECTION('',(1.,0.,0.));
#32161=DIRECTION('',(0.577350269189616,-0.577350269189646,0.577350269189616));
#32162=DIRECTION('',(-0.577350269189616,-0.577350269189646,0.577350269189616));
#32163=DIRECTION('center_axis',(0.707106781186566,-0.707106781186529,0.));
#32164=DIRECTION('ref_axis',(0.,0.,-1.));
#32165=DIRECTION('',(-0.577350269189616,-0.577350269189646,-0.577350269189616));
#32166=DIRECTION('',(0.,0.,1.));
#32167=DIRECTION('',(0.577350269189616,0.577350269189646,-0.577350269189616));
#32168=DIRECTION('center_axis',(0.707106781186548,0.,-0.707106781186548));
#32169=DIRECTION('ref_axis',(-0.707106781186548,0.,-0.707106781186548));
#32170=DIRECTION('',(0.,1.,0.));
#32171=DIRECTION('',(-0.577350269189616,-0.577350269189646,-0.577350269189616));
#32172=DIRECTION('',(0.,-1.,0.));
#32173=DIRECTION('center_axis',(-0.707106781186566,0.707106781186529,0.));
#32174=DIRECTION('ref_axis',(0.,0.,1.));
#32175=DIRECTION('',(0.,0.,-1.));
#32176=DIRECTION('',(0.577350269189616,0.577350269189646,0.577350269189616));
#32177=DIRECTION('',(0.577350269189616,0.577350269189646,-0.577350269189616));
#32178=DIRECTION('',(0.,0.,1.));
#32179=DIRECTION('center_axis',(0.,1.,0.));
#32180=DIRECTION('ref_axis',(0.,0.,1.));
#32181=DIRECTION('',(0.,0.,1.));
#32182=DIRECTION('',(1.,0.,0.));
#32183=DIRECTION('',(0.,0.,1.));
#32184=DIRECTION('',(1.,0.,0.));
#32185=DIRECTION('',(0.,0.,-1.));
#32186=DIRECTION('',(1.,0.,0.));
#32187=DIRECTION('center_axis',(0.,0.707106781186529,-0.707106781186566));
#32188=DIRECTION('ref_axis',(-1.,0.,0.));
#32189=DIRECTION('',(0.577350269189643,0.577350269189633,0.577350269189602));
#32190=DIRECTION('',(-1.,0.,0.));
#32191=DIRECTION('',(-0.577350269189616,0.577350269189646,0.577350269189616));
#32192=DIRECTION('center_axis',(-0.707106781186548,0.,-0.707106781186548));
#32193=DIRECTION('ref_axis',(-0.707106781186548,0.,0.707106781186548));
#32194=DIRECTION('',(0.,-1.,0.));
#32195=DIRECTION('',(-0.707106781186548,0.,0.707106781186548));
#32196=DIRECTION('',(0.,1.,0.));
#32197=DIRECTION('center_axis',(-0.707106781186554,-0.707106781186541,0.));
#32198=DIRECTION('ref_axis',(0.,0.,1.));
#32199=DIRECTION('',(-0.577350269189613,0.577350269189624,-0.577350269189641));
#32200=DIRECTION('',(0.,0.,-1.));
#32201=DIRECTION('center_axis',(0.,0.,1.));
#32202=DIRECTION('ref_axis',(0.,-1.,0.));
#32203=DIRECTION('',(0.,1.,0.));
#32204=DIRECTION('',(1.,0.,0.));
#32205=DIRECTION('center_axis',(-1.,0.,0.));
#32206=DIRECTION('ref_axis',(0.,-1.,0.));
#32207=DIRECTION('',(0.,-1.,0.));
#32208=DIRECTION('',(0.,0.,1.));
#32209=DIRECTION('',(0.,1.,0.));
#32210=DIRECTION('',(0.,-0.707106781186566,-0.707106781186529));
#32211=DIRECTION('',(0.,0.,-1.));
#32212=DIRECTION('',(0.,1.,0.));
#32213=DIRECTION('',(0.,0.,-1.));
#32214=DIRECTION('',(0.,-0.707106781186566,0.707106781186529));
#32215=DIRECTION('center_axis',(-0.707106781186564,0.,0.707106781186531));
#32216=DIRECTION('ref_axis',(0.707106781186531,0.,0.707106781186564));
#32217=DIRECTION('',(0.,1.,0.));
#32218=DIRECTION('',(-0.577350269189614,0.577350269189621,-0.577350269189642));
#32219=DIRECTION('',(0.57735026918962,0.57735026918961,0.577350269189647));
#32220=DIRECTION('center_axis',(-0.577350269189636,-0.577350269189605,-0.577350269189636));
#32221=DIRECTION('ref_axis',(-0.707106781186548,0.,0.707106781186548));
#32222=DIRECTION('',(0.,0.707106781186566,-0.707106781186529));
#32223=DIRECTION('',(0.707106781186529,-0.707106781186566,0.));
#32224=DIRECTION('center_axis',(-0.707106781186566,-0.707106781186529,0.));
#32225=DIRECTION('ref_axis',(0.,0.,1.));
#32226=DIRECTION('',(-0.577350269189616,0.577350269189646,-0.577350269189616));
#32227=DIRECTION('',(0.,0.,-1.));
#32228=DIRECTION('',(0.,0.,1.));
#32229=DIRECTION('',(-0.577350269189616,0.577350269189646,0.577350269189616));
#32230=DIRECTION('center_axis',(0.,-0.707106781186529,-0.707106781186566));
#32231=DIRECTION('ref_axis',(-1.,0.,0.));
#32232=DIRECTION('',(0.,0.707106781186566,-0.707106781186529));
#32233=DIRECTION('',(-1.,0.,0.));
#32234=DIRECTION('',(1.,0.,0.));
#32235=DIRECTION('center_axis',(1.,0.,0.));
#32236=DIRECTION('ref_axis',(0.,0.,-1.));
#32237=DIRECTION('',(0.,-1.,0.));
#32238=DIRECTION('',(0.,0.,1.));
#32239=DIRECTION('center_axis',(-0.707106781186548,0.,0.707106781186548));
#32240=DIRECTION('ref_axis',(0.707106781186548,0.,0.707106781186548));
#32241=DIRECTION('',(0.577350269189616,0.577350269189646,0.577350269189616));
#32242=DIRECTION('',(0.,1.,0.));
#32243=DIRECTION('',(0.577350269189616,-0.577350269189646,0.577350269189616));
#32244=DIRECTION('',(-0.577350269189616,-0.577350269189646,-0.577350269189616));
#32245=DIRECTION('center_axis',(0.,-0.707106781186529,0.707106781186566));
#32246=DIRECTION('ref_axis',(1.,0.,0.));
#32247=DIRECTION('',(1.,0.,0.));
#32248=DIRECTION('',(-1.,0.,0.));
#32249=DIRECTION('center_axis',(0.,-1.,0.));
#32250=DIRECTION('ref_axis',(0.,0.,-1.));
#32251=DIRECTION('',(0.,0.,-1.));
#32252=DIRECTION('',(0.707106781186573,0.,0.707106781186522));
#32253=DIRECTION('',(1.,0.,0.));
#32254=DIRECTION('',(0.707106781186573,0.,-0.707106781186522));
#32255=DIRECTION('',(0.,0.,-1.));
#32256=DIRECTION('',(-1.,0.,0.));
#32257=DIRECTION('',(0.,0.,-1.));
#32258=DIRECTION('',(1.,0.,0.));
#32259=DIRECTION('',(0.,0.,1.));
#32260=DIRECTION('',(-0.707106781186573,0.,-0.707106781186522));
#32261=DIRECTION('',(1.,0.,0.));
#32262=DIRECTION('',(-0.707106781186573,0.,0.707106781186522));
#32263=DIRECTION('center_axis',(0.,-0.707106781186529,0.707106781186566));
#32264=DIRECTION('ref_axis',(1.,0.,0.));
#32265=DIRECTION('',(-0.577350269189616,0.577350269189646,0.577350269189616));
#32266=DIRECTION('',(-1.,0.,0.));
#32267=DIRECTION('',(0.,0.707106781186566,0.707106781186529));
#32268=DIRECTION('',(0.577350269189616,0.577350269189646,0.577350269189616));
#32269=DIRECTION('center_axis',(0.707106781186548,0.,0.707106781186548));
#32270=DIRECTION('ref_axis',(0.707106781186548,0.,-0.707106781186548));
#32271=DIRECTION('',(-0.577350269189616,-0.577350269189646,0.577350269189616));
#32272=DIRECTION('',(0.,1.,0.));
#32273=DIRECTION('',(-0.577350269189616,0.577350269189646,0.577350269189616));
#32274=DIRECTION('',(-0.577350269189616,-0.577350269189646,0.577350269189616));
#32275=DIRECTION('',(0.,-1.,0.));
#32276=DIRECTION('center_axis',(0.707106781186566,-0.707106781186529,0.));
#32277=DIRECTION('ref_axis',(0.,0.,-1.));
#32278=DIRECTION('',(-0.577350269189616,-0.577350269189646,0.577350269189616));
#32279=DIRECTION('',(-0.577350269189616,-0.577350269189646,-0.577350269189616));
#32280=DIRECTION('',(0.,0.,1.));
#32281=DIRECTION('center_axis',(0.,0.707106781186529,-0.707106781186566));
#32282=DIRECTION('ref_axis',(-1.,0.,0.));
#32283=DIRECTION('',(0.577350269189616,-0.577350269189646,-0.577350269189616));
#32284=DIRECTION('',(-0.577350269189616,-0.577350269189646,-0.577350269189616));
#32285=DIRECTION('',(-1.,0.,0.));
#32286=DIRECTION('',(-0.577350269189616,0.577350269189646,0.577350269189616));
#32287=DIRECTION('center_axis',(0.707106781186554,0.707106781186541,0.));
#32288=DIRECTION('ref_axis',(0.,0.,-1.));
#32289=DIRECTION('',(0.,0.,-1.));
#32290=DIRECTION('',(-0.577350269189613,0.577350269189624,-0.577350269189641));
#32291=DIRECTION('',(-0.577350269189612,0.577350269189622,0.577350269189643));
#32292=DIRECTION('center_axis',(0.707106781186566,0.707106781186529,0.));
#32293=DIRECTION('ref_axis',(0.,0.,-1.));
#32294=DIRECTION('',(-0.577350269189616,0.577350269189646,0.577350269189616));
#32295=DIRECTION('',(0.,0.,-1.));
#32296=DIRECTION('',(0.577350269189616,-0.577350269189646,0.577350269189616));
#32297=DIRECTION('center_axis',(0.,0.70710678118656,-0.707106781186535));
#32298=DIRECTION('ref_axis',(-1.,0.,0.));
#32299=DIRECTION('',(0.577350269189605,0.577350269189626,0.577350269189646));
#32300=DIRECTION('',(-1.,0.,0.));
#32301=DIRECTION('',(0.577350269189614,-0.577350269189621,-0.577350269189642));
#32302=DIRECTION('',(-0.577350269189626,-0.577350269189615,-0.577350269189636));
#32303=DIRECTION('center_axis',(0.707106781186522,0.,0.707106781186573));
#32304=DIRECTION('ref_axis',(0.707106781186573,0.,-0.707106781186522));
#32305=DIRECTION('',(-0.707106781186573,0.,0.707106781186522));
#32306=DIRECTION('',(0.,1.,0.));
#32307=DIRECTION('',(0.,-1.,0.));
#32308=DIRECTION('center_axis',(1.,0.,0.));
#32309=DIRECTION('ref_axis',(0.,1.,0.));
#32310=DIRECTION('',(0.,1.,0.));
#32311=DIRECTION('',(0.,-0.707106781186566,0.707106781186529));
#32312=DIRECTION('',(0.,0.,1.));
#32313=DIRECTION('',(0.,-0.707106781186566,-0.707106781186529));
#32314=DIRECTION('',(0.,1.,0.));
#32315=DIRECTION('',(0.,0.,1.));
#32316=DIRECTION('',(0.,-1.,0.));
#32317=DIRECTION('center_axis',(0.,-0.707106781186529,-0.707106781186566));
#32318=DIRECTION('ref_axis',(-1.,0.,0.));
#32319=DIRECTION('',(1.,0.,0.));
#32320=DIRECTION('',(0.577350269189616,-0.577350269189646,0.577350269189616));
#32321=DIRECTION('center_axis',(0.707106781186548,0.,-0.707106781186548));
#32322=DIRECTION('ref_axis',(-0.707106781186548,0.,-0.707106781186548));
#32323=DIRECTION('',(0.,-1.,0.));
#32324=DIRECTION('',(0.,1.,0.));
#32325=DIRECTION('center_axis',(0.707106781186548,0.,-0.707106781186548));
#32326=DIRECTION('ref_axis',(-0.707106781186548,0.,-0.707106781186548));
#32327=DIRECTION('',(0.577350269189616,-0.577350269189646,0.577350269189616));
#32328=DIRECTION('',(0.,-1.,0.));
#32329=DIRECTION('',(-0.577350269189616,0.577350269189646,-0.577350269189616));
#32330=DIRECTION('center_axis',(0.707106781186566,0.707106781186529,0.));
#32331=DIRECTION('ref_axis',(0.,0.,-1.));
#32332=DIRECTION('',(0.,0.,-1.));
#32333=DIRECTION('',(-0.577350269189616,0.577350269189646,0.577350269189616));
#32334=DIRECTION('center_axis',(0.707106781186548,0.,0.707106781186548));
#32335=DIRECTION('ref_axis',(0.707106781186548,0.,-0.707106781186548));
#32336=DIRECTION('',(0.,1.,0.));
#32337=DIRECTION('center_axis',(1.,0.,0.));
#32338=DIRECTION('ref_axis',(0.,0.,-1.));
#32339=DIRECTION('',(0.,0.,-1.));
#32340=DIRECTION('center_axis',(0.707106781186566,0.707106781186529,0.));
#32341=DIRECTION('ref_axis',(0.,0.,-1.));
#32342=DIRECTION('',(0.,0.,1.));
#32343=DIRECTION('',(-0.577350269189616,0.577350269189646,-0.577350269189616));
#32344=DIRECTION('center_axis',(0.,0.,-1.));
#32345=DIRECTION('ref_axis',(0.,1.,0.));
#32346=DIRECTION('center_axis',(0.,0.,1.));
#32347=DIRECTION('ref_axis',(0.,-1.,0.));
#32348=DIRECTION('',(1.,0.,0.));
#32349=DIRECTION('',(0.,-1.,0.));
#32350=DIRECTION('center_axis',(0.,0.707106781186529,0.707106781186566));
#32351=DIRECTION('ref_axis',(1.,0.,0.));
#32352=DIRECTION('',(-1.,0.,0.));
#32353=DIRECTION('',(0.577350269189616,-0.577350269189646,0.577350269189616));
#32354=DIRECTION('center_axis',(0.,1.,0.));
#32355=DIRECTION('ref_axis',(0.,0.,1.));
#32356=DIRECTION('',(0.,0.,-1.));
#32357=DIRECTION('',(-1.,0.,0.));
#32358=DIRECTION('',(0.,0.,-1.));
#32359=DIRECTION('',(-1.,0.,0.));
#32360=DIRECTION('',(0.,0.,1.));
#32361=DIRECTION('center_axis',(0.707106781186554,0.707106781186541,0.));
#32362=DIRECTION('ref_axis',(0.,0.,-1.));
#32363=DIRECTION('',(0.577350269189612,-0.577350269189622,0.577350269189643));
#32364=DIRECTION('',(0.,0.,-1.));
#32365=DIRECTION('center_axis',(0.,0.70710678118656,0.707106781186535));
#32366=DIRECTION('ref_axis',(1.,0.,0.));
#32367=DIRECTION('',(0.577350269189626,0.577350269189615,-0.577350269189636));
#32368=DIRECTION('',(1.,0.,0.));
#32369=DIRECTION('center_axis',(-0.707106781186541,0.707106781186554,0.));
#32370=DIRECTION('ref_axis',(0.,0.,1.));
#32371=DIRECTION('',(-0.577350269189629,-0.577350269189639,0.577350269189609));
#32372=DIRECTION('center_axis',(0.,0.707106781186529,0.707106781186566));
#32373=DIRECTION('ref_axis',(1.,0.,0.));
#32374=DIRECTION('',(-0.577350269189616,-0.577350269189646,0.577350269189616));
#32375=DIRECTION('',(1.,0.,0.));
#32376=DIRECTION('center_axis',(0.,0.,1.));
#32377=DIRECTION('ref_axis',(0.,-1.,0.));
#32378=DIRECTION('center_axis',(-0.707106781186541,0.707106781186554,0.));
#32379=DIRECTION('ref_axis',(0.,0.,1.));
#32380=DIRECTION('',(-0.57735026918962,-0.57735026918961,0.577350269189647));
#32381=DIRECTION('',(0.,0.,1.));
#32382=DIRECTION('center_axis',(-0.707106781186522,0.,0.707106781186573));
#32383=DIRECTION('ref_axis',(0.707106781186573,0.,0.707106781186522));
#32384=DIRECTION('',(0.,-1.,0.));
#32385=DIRECTION('',(-0.707106781186573,0.,-0.707106781186522));
#32386=DIRECTION('',(0.,1.,0.));
#32387=DIRECTION('center_axis',(-1.,0.,0.));
#32388=DIRECTION('ref_axis',(0.,-1.,0.));
#32389=DIRECTION('',(0.,1.,0.));
#32390=DIRECTION('',(0.,0.,-1.));
#32391=DIRECTION('',(0.,-1.,0.));
#32392=DIRECTION('',(0.,0.707106781186566,0.707106781186529));
#32393=DIRECTION('',(0.,0.,-1.));
#32394=DIRECTION('',(0.,-1.,0.));
#32395=DIRECTION('center_axis',(0.707106781186522,0.,-0.707106781186573));
#32396=DIRECTION('ref_axis',(-0.707106781186573,0.,-0.707106781186522));
#32397=DIRECTION('',(0.,-1.,0.));
#32398=DIRECTION('',(0.707106781186573,0.,0.707106781186522));
#32399=DIRECTION('',(0.,1.,0.));
#32400=DIRECTION('center_axis',(0.,0.,1.));
#32401=DIRECTION('ref_axis',(1.,0.,0.));
#32402=DIRECTION('',(1.,0.,0.));
#32403=DIRECTION('',(0.,-1.,0.));
#32404=DIRECTION('center_axis',(0.,0.,-1.));
#32405=DIRECTION('ref_axis',(1.,0.,0.));
#32406=DIRECTION('center_axis',(0.,0.,-1.));
#32407=DIRECTION('ref_axis',(1.,0.,0.));
#32408=DIRECTION('center_axis',(0.,0.707106781186529,0.707106781186566));
#32409=DIRECTION('ref_axis',(1.,0.,0.));
#32410=DIRECTION('',(-0.577350269189616,0.577350269189646,-0.577350269189616));
#32411=DIRECTION('',(-1.,0.,0.));
#32412=DIRECTION('',(0.,0.707106781186566,-0.707106781186529));
#32413=DIRECTION('',(1.,0.,0.));
#32414=DIRECTION('',(0.577350269189616,0.577350269189646,-0.577350269189616));
#32415=DIRECTION('center_axis',(0.,1.,0.));
#32416=DIRECTION('ref_axis',(0.,0.,1.));
#32417=DIRECTION('',(0.,0.,1.));
#32418=DIRECTION('',(0.,0.,1.));
#32419=DIRECTION('',(1.,0.,0.));
#32420=DIRECTION('',(1.,0.,0.));
#32421=DIRECTION('',(1.,0.,0.));
#32422=DIRECTION('',(0.,0.,-1.));
#32423=DIRECTION('',(-1.,0.,0.));
#32424=DIRECTION('',(0.707106781186573,0.,-0.707106781186522));
#32425=DIRECTION('center_axis',(0.707106781186566,0.707106781186529,0.));
#32426=DIRECTION('ref_axis',(0.,0.,-1.));
#32427=DIRECTION('',(-0.577350269189616,0.577350269189646,0.577350269189616));
#32428=DIRECTION('',(0.,0.,-1.));
#32429=DIRECTION('',(-0.707106781186529,0.707106781186566,0.));
#32430=DIRECTION('center_axis',(0.707106781186548,0.,0.707106781186548));
#32431=DIRECTION('ref_axis',(0.707106781186548,0.,-0.707106781186548));
#32432=DIRECTION('',(0.,1.,0.));
#32433=DIRECTION('',(0.,-1.,0.));
#32434=DIRECTION('center_axis',(-0.707106781186566,0.707106781186529,0.));
#32435=DIRECTION('ref_axis',(0.,0.,1.));
#32436=DIRECTION('center_axis',(-0.707106781186522,0.,-0.707106781186573));
#32437=DIRECTION('ref_axis',(-0.707106781186573,0.,0.707106781186522));
#32438=DIRECTION('center_axis',(-0.707106781186541,0.707106781186554,0.));
#32439=DIRECTION('ref_axis',(0.,0.,1.));
#32440=DIRECTION('',(0.577350269189643,0.577350269189633,-0.577350269189602));
#32441=DIRECTION('',(-0.577350269189643,-0.577350269189633,-0.577350269189602));
#32442=DIRECTION('',(-0.577350269189643,-0.577350269189633,0.577350269189602));
#32443=DIRECTION('center_axis',(0.,0.707106781186529,0.707106781186566));
#32444=DIRECTION('ref_axis',(1.,0.,0.));
#32445=DIRECTION('center_axis',(0.,0.707106781186529,-0.707106781186566));
#32446=DIRECTION('ref_axis',(-1.,0.,0.));
#32447=DIRECTION('',(-1.,0.,0.));
#32448=DIRECTION('',(0.577350269189643,-0.577350269189633,-0.577350269189602));
#32449=DIRECTION('center_axis',(0.707106781186548,0.,0.707106781186548));
#32450=DIRECTION('ref_axis',(0.707106781186548,0.,-0.707106781186548));
#32451=DIRECTION('',(0.577350269189616,0.577350269189646,-0.577350269189616));
#32452=DIRECTION('',(0.,1.,0.));
#32453=DIRECTION('',(-0.577350269189616,-0.577350269189646,0.577350269189616));
#32454=DIRECTION('center_axis',(0.707106781186566,-0.707106781186529,0.));
#32455=DIRECTION('ref_axis',(0.,0.,-1.));
#32456=DIRECTION('',(0.,0.,1.));
#32457=DIRECTION('center_axis',(1.,0.,0.));
#32458=DIRECTION('ref_axis',(0.,0.,-1.));
#32459=DIRECTION('',(0.,0.,1.));
#32460=DIRECTION('',(0.,-1.,0.));
#32461=DIRECTION('center_axis',(0.707106781186566,-0.707106781186529,0.));
#32462=DIRECTION('ref_axis',(0.,0.,-1.));
#32463=DIRECTION('',(0.,0.,-1.));
#32464=DIRECTION('',(-0.577350269189616,-0.577350269189646,0.577350269189616));
#32465=DIRECTION('',(-0.577350269189616,-0.577350269189646,-0.577350269189616));
#32466=DIRECTION('center_axis',(0.577350269189636,0.577350269189605,-0.577350269189636));
#32467=DIRECTION('ref_axis',(-0.707106781186548,0.,-0.707106781186548));
#32468=DIRECTION('',(0.707106781186548,0.,0.707106781186548));
#32469=DIRECTION('',(0.,-0.707106781186566,-0.707106781186529));
#32470=DIRECTION('center_axis',(0.,0.707106781186529,-0.707106781186566));
#32471=DIRECTION('ref_axis',(-1.,0.,0.));
#32472=DIRECTION('',(-1.,0.,0.));
#32473=DIRECTION('center_axis',(0.707106781186548,0.,-0.707106781186548));
#32474=DIRECTION('ref_axis',(-0.707106781186548,0.,-0.707106781186548));
#32475=DIRECTION('',(-0.577350269189616,0.577350269189646,-0.577350269189616));
#32476=DIRECTION('',(0.,1.,0.));
#32477=DIRECTION('center_axis',(0.,0.,-1.));
#32478=DIRECTION('ref_axis',(0.,1.,0.));
#32479=DIRECTION('',(1.,0.,0.));
#32480=DIRECTION('center_axis',(0.,-0.707106781186529,-0.707106781186566));
#32481=DIRECTION('ref_axis',(-1.,0.,0.));
#32482=DIRECTION('',(-1.,0.,0.));
#32483=DIRECTION('',(0.577350269189616,0.577350269189646,-0.577350269189616));
#32484=DIRECTION('center_axis',(-0.707106781186522,0.,-0.707106781186573));
#32485=DIRECTION('ref_axis',(-0.707106781186573,0.,0.707106781186522));
#32486=DIRECTION('',(0.,-1.,0.));
#32487=DIRECTION('',(-0.577350269189643,-0.577350269189633,0.577350269189602));
#32488=DIRECTION('',(-0.577350269189643,0.577350269189633,0.577350269189602));
#32489=DIRECTION('center_axis',(0.,-0.707106781186529,-0.707106781186566));
#32490=DIRECTION('ref_axis',(-1.,0.,0.));
#32491=DIRECTION('',(1.,0.,0.));
#32492=DIRECTION('',(-0.577350269189616,0.577350269189646,-0.577350269189616));
#32493=DIRECTION('',(-1.,0.,0.));
#32494=DIRECTION('',(-0.577350269189643,0.577350269189633,-0.577350269189602));
#32495=DIRECTION('center_axis',(0.,0.,-1.));
#32496=DIRECTION('ref_axis',(0.,1.,0.));
#32497=DIRECTION('center_axis',(0.,-1.,0.));
#32498=DIRECTION('ref_axis',(0.,0.,-1.));
#32499=DIRECTION('',(0.,0.,1.));
#32500=DIRECTION('',(0.,0.,1.));
#32501=DIRECTION('',(-1.,0.,0.));
#32502=DIRECTION('',(0.,0.,-1.));
#32503=DIRECTION('center_axis',(0.707106781186554,-0.707106781186541,0.));
#32504=DIRECTION('ref_axis',(0.,0.,-1.));
#32505=DIRECTION('',(0.577350269189612,0.577350269189622,-0.577350269189643));
#32506=DIRECTION('',(0.577350269189613,0.577350269189624,0.577350269189641));
#32507=DIRECTION('center_axis',(0.707106781186564,0.,-0.707106781186531));
#32508=DIRECTION('ref_axis',(-0.707106781186531,0.,-0.707106781186564));
#32509=DIRECTION('',(0.577350269189614,-0.577350269189621,0.577350269189642));
#32510=DIRECTION('',(0.,1.,0.));
#32511=DIRECTION('center_axis',(0.,-0.70710678118656,-0.707106781186535));
#32512=DIRECTION('ref_axis',(-1.,0.,0.));
#32513=DIRECTION('',(0.577350269189612,-0.577350269189622,0.577350269189643));
#32514=DIRECTION('',(-0.577350269189614,-0.577350269189621,0.577350269189642));
#32515=DIRECTION('',(1.,0.,0.));
#32516=DIRECTION('center_axis',(-0.707106781186554,-0.707106781186541,0.));
#32517=DIRECTION('ref_axis',(0.,0.,1.));
#32518=DIRECTION('',(0.577350269189613,-0.577350269189624,-0.577350269189641));
#32519=DIRECTION('center_axis',(-0.707106781186564,0.,-0.707106781186531));
#32520=DIRECTION('ref_axis',(-0.707106781186531,0.,0.707106781186564));
#32521=DIRECTION('',(0.,-1.,0.));
#32522=DIRECTION('center_axis',(-0.707106781186541,-0.707106781186554,0.));
#32523=DIRECTION('ref_axis',(0.,0.,1.));
#32524=DIRECTION('center_axis',(0.,8.71363591613481E-16,1.));
#32525=DIRECTION('ref_axis',(-1.,-3.01769808787504E-17,0.));
#32526=DIRECTION('center_axis',(0.,0.,-1.));
#32527=DIRECTION('ref_axis',(-1.,0.,0.));
#32528=DIRECTION('center_axis',(0.,0.,-1.));
#32529=DIRECTION('ref_axis',(-1.,0.,0.));
#32530=DIRECTION('',(-0.382683432365075,-8.63448422341581E-16,-0.923879532511293));
#32531=DIRECTION('center_axis',(0.,0.,1.));
#32532=DIRECTION('ref_axis',(-1.,-6.12323399573677E-17,0.));
#32533=DIRECTION('center_axis',(0.,0.,1.));
#32534=DIRECTION('ref_axis',(-1.,-6.12323399573677E-17,0.));
#32535=DIRECTION('center_axis',(0.,0.,1.));
#32536=DIRECTION('ref_axis',(1.,0.,0.));
#32537=DIRECTION('',(0.707106781186543,8.65956056235488E-17,-0.707106781186552));
#32538=DIRECTION('center_axis',(0.,0.,-1.));
#32539=DIRECTION('ref_axis',(-1.,-6.12323399573677E-17,0.));
#32540=DIRECTION('center_axis',(0.,0.,-1.));
#32541=DIRECTION('ref_axis',(-1.,-6.12323399573677E-17,0.));
#32542=DIRECTION('center_axis',(0.,0.,1.));
#32543=DIRECTION('ref_axis',(1.,0.,0.));
#32544=DIRECTION('center_axis',(0.,0.,1.));
#32545=DIRECTION('ref_axis',(1.,0.,0.));
#32546=DIRECTION('',(0.,0.,-1.));
#32547=DIRECTION('center_axis',(0.,-2.05293126929891E-15,1.));
#32548=DIRECTION('ref_axis',(-1.,-3.17596479860489E-17,0.));
#32549=DIRECTION('',(-0.923879532511284,6.43138084582096E-16,-0.382683432365096));
#32550=DIRECTION('center_axis',(0.,0.,1.));
#32551=DIRECTION('ref_axis',(-1.,0.,0.));
#32552=DIRECTION('center_axis',(0.,0.,-1.));
#32553=DIRECTION('ref_axis',(-1.,0.,0.));
#32554=DIRECTION('center_axis',(0.,0.,-1.));
#32555=DIRECTION('ref_axis',(1.,0.,0.));
#32556=DIRECTION('',(0.707106781186573,-8.65956056235524E-17,0.707106781186522));
#32557=DIRECTION('center_axis',(0.,0.,1.));
#32558=DIRECTION('ref_axis',(1.,0.,0.));
#32559=DIRECTION('center_axis',(0.,0.,1.));
#32560=DIRECTION('ref_axis',(1.,0.,0.));
#32561=DIRECTION('',(0.,0.,1.));
#32562=DIRECTION('center_axis',(0.,0.,-1.));
#32563=DIRECTION('ref_axis',(1.,0.,0.));
#32564=DIRECTION('center_axis',(0.,0.,1.));
#32565=DIRECTION('ref_axis',(1.,0.,0.));
#32566=DIRECTION('center_axis',(0.,0.,1.));
#32567=DIRECTION('ref_axis',(1.,0.,0.));
#32568=DIRECTION('',(0.707106781186573,8.65956056235524E-17,-0.707106781186522));
#32569=DIRECTION('center_axis',(0.,0.,1.));
#32570=DIRECTION('ref_axis',(1.,0.,0.));
#32571=DIRECTION('center_axis',(0.,0.,1.));
#32572=DIRECTION('ref_axis',(1.,0.,0.));
#32573=DIRECTION('center_axis',(0.,0.,-1.));
#32574=DIRECTION('ref_axis',(1.,0.,0.));
#32575=DIRECTION('',(0.707106781186573,-8.65956056235524E-17,0.707106781186522));
#32576=DIRECTION('center_axis',(0.,0.,1.));
#32577=DIRECTION('ref_axis',(1.,0.,0.));
#32578=DIRECTION('center_axis',(0.,0.,1.));
#32579=DIRECTION('ref_axis',(1.,0.,0.));
#32580=DIRECTION('',(0.,0.,1.));
#32581=DIRECTION('center_axis',(0.,0.,-1.));
#32582=DIRECTION('ref_axis',(1.,0.,0.));
#32583=DIRECTION('center_axis',(0.,0.,1.));
#32584=DIRECTION('ref_axis',(1.,0.,0.));
#32585=DIRECTION('',(0.707106781186573,8.65956056235524E-17,-0.707106781186522));
#32586=DIRECTION('center_axis',(0.,0.,1.));
#32587=DIRECTION('ref_axis',(1.,0.,0.));
#32588=DIRECTION('center_axis',(0.,0.,1.));
#32589=DIRECTION('ref_axis',(1.,0.,0.));
#32590=DIRECTION('',(0.650791373455974,7.96989572415569E-17,-0.759256602365292));
#32591=DIRECTION('center_axis',(0.,0.,-1.));
#32592=DIRECTION('ref_axis',(0.,1.,0.));
#32593=DIRECTION('center_axis',(0.,0.,-1.));
#32594=DIRECTION('ref_axis',(0.,1.,0.));
#32595=DIRECTION('center_axis',(0.,0.,1.));
#32596=DIRECTION('ref_axis',(1.,0.,0.));
#32597=DIRECTION('center_axis',(0.,0.,1.));
#32598=DIRECTION('ref_axis',(1.,0.,0.));
#32599=DIRECTION('center_axis',(1.,0.,0.));
#32600=DIRECTION('ref_axis',(0.,1.,0.));
#32601=DIRECTION('',(0.,-1.,0.));
#32602=DIRECTION('center_axis',(0.,0.,1.));
#32603=DIRECTION('ref_axis',(0.,-1.,0.));
#42153=CARTESIAN_POINT('',(0.,0.,0.));
#42154=CARTESIAN_POINT('Origin',(-37.95,-4.65,103.7));
#42155=CARTESIAN_POINT('',(-37.9,-4.7,98.6));
#42156=CARTESIAN_POINT('',(-37.9,-4.7,105.4));
#42157=CARTESIAN_POINT('',(-37.9,-4.7,103.7));
#42158=CARTESIAN_POINT('',(-38.,-4.6,105.5));
#42159=CARTESIAN_POINT('',(-37.1875,-5.41250000000001,104.6875));
#42160=CARTESIAN_POINT('',(-38.,-4.6,98.5));
#42161=CARTESIAN_POINT('',(-38.,-4.6,103.7));
#42162=CARTESIAN_POINT('',(-38.,-4.6,98.5));
#42163=CARTESIAN_POINT('Origin',(-37.95,-5.525,98.55));
#42164=CARTESIAN_POINT('',(-38.,-8.5,98.5));
#42165=CARTESIAN_POINT('',(-38.,-5.525,98.5));
#42166=CARTESIAN_POINT('',(-37.95,-8.55,98.55));
#42167=CARTESIAN_POINT('',(-38.1625,-8.33749999999998,98.3375));
#42168=CARTESIAN_POINT('',(-37.9,-8.5,98.6));
#42169=CARTESIAN_POINT('',(-37.4541666666667,-8.05416666666666,99.0458333333333));
#42170=CARTESIAN_POINT('',(-37.9,-5.525,98.6));
#42171=CARTESIAN_POINT('Origin',(-38.,-4.7,105.4));
#42172=CARTESIAN_POINT('',(37.9,-4.7,98.6));
#42173=CARTESIAN_POINT('',(-38.,-4.7,98.6));
#42174=CARTESIAN_POINT('',(37.9,-4.7,105.4));
#42175=CARTESIAN_POINT('',(37.9,-4.7,103.7));
#42176=CARTESIAN_POINT('',(-38.,-4.7,105.4));
#42177=CARTESIAN_POINT('Origin',(-38.,-4.7,98.6));
#42178=CARTESIAN_POINT('',(37.9,-8.5,98.6));
#42179=CARTESIAN_POINT('',(-38.,-8.5,98.6));
#42180=CARTESIAN_POINT('',(37.9,-5.525,98.6));
#42181=CARTESIAN_POINT('Origin',(-38.,-8.55,98.55));
#42182=CARTESIAN_POINT('',(-37.9,-8.6,98.5));
#42183=CARTESIAN_POINT('',(-38.25,-8.25000000000001,98.85));
#42184=CARTESIAN_POINT('',(37.9,-8.6,98.5));
#42185=CARTESIAN_POINT('',(-38.,-8.6,98.5));
#42186=CARTESIAN_POINT('',(37.95,-8.55,98.55));
#42187=CARTESIAN_POINT('',(25.5833333333338,-20.9166666666669,86.1833333333338));
#42188=CARTESIAN_POINT('',(24.7875000000004,4.61250000000026,111.7125));
#42189=CARTESIAN_POINT('Origin',(-37.95,7.475,98.55));
#42190=CARTESIAN_POINT('',(-37.9,4.7,98.6));
#42191=CARTESIAN_POINT('',(-37.9,8.5,98.6));
#42192=CARTESIAN_POINT('',(-37.9,7.475,98.6));
#42193=CARTESIAN_POINT('',(-37.95,8.55,98.55));
#42194=CARTESIAN_POINT('',(-37.7791666666667,8.37916666666666,98.7208333333333));
#42195=CARTESIAN_POINT('',(-38.,8.5,98.5));
#42196=CARTESIAN_POINT('',(-37.8875,8.61249999999999,98.6125));
#42197=CARTESIAN_POINT('',(-38.,4.6,98.5));
#42198=CARTESIAN_POINT('',(-38.,7.475,98.5));
#42199=CARTESIAN_POINT('',(-38.,4.6,98.5));
#42200=CARTESIAN_POINT('Origin',(-37.95,4.65,100.3));
#42201=CARTESIAN_POINT('',(-37.9,4.7,105.4));
#42202=CARTESIAN_POINT('',(-37.9,4.7,100.3));
#42203=CARTESIAN_POINT('',(-38.,4.6,105.5));
#42204=CARTESIAN_POINT('',(-38.,4.6,100.3));
#42205=CARTESIAN_POINT('',(-38.,4.6,105.5));
#42206=CARTESIAN_POINT('Origin',(-37.95,5.525,105.45));
#42207=CARTESIAN_POINT('',(-38.,8.5,105.5));
#42208=CARTESIAN_POINT('',(-38.,5.525,105.5));
#42209=CARTESIAN_POINT('',(-37.95,8.55,105.45));
#42210=CARTESIAN_POINT('',(-38.1625,8.33749999999997,105.6625));
#42211=CARTESIAN_POINT('',(-37.9,8.5,105.4));
#42212=CARTESIAN_POINT('',(-37.4541666666667,8.05416666666663,104.954166666667));
#42213=CARTESIAN_POINT('',(-37.9,5.525,105.4));
#42214=CARTESIAN_POINT('Origin',(-38.,8.55,98.55));
#42215=CARTESIAN_POINT('',(37.9,8.5,98.6));
#42216=CARTESIAN_POINT('',(-38.,8.5,98.6));
#42217=CARTESIAN_POINT('',(37.95,8.54999999999999,98.55));
#42218=CARTESIAN_POINT('',(25.1125000000005,-4.28750000000024,111.3875));
#42219=CARTESIAN_POINT('',(37.9,8.6,98.5));
#42220=CARTESIAN_POINT('',(25.5333333333338,20.9666666666669,86.1333333333338));
#42221=CARTESIAN_POINT('',(-37.9,8.6,98.5));
#42222=CARTESIAN_POINT('',(-38.,8.6,98.5));
#42223=CARTESIAN_POINT('',(-38.2,8.3,98.8));
#42224=CARTESIAN_POINT('Origin',(-38.,8.6,98.6));
#42225=CARTESIAN_POINT('',(37.9,4.7,98.6));
#42226=CARTESIAN_POINT('',(-38.,4.7,98.6));
#42227=CARTESIAN_POINT('',(37.9,7.475,98.6));
#42228=CARTESIAN_POINT('Origin',(-38.,4.7,98.6));
#42229=CARTESIAN_POINT('',(37.9,4.7,105.4));
#42230=CARTESIAN_POINT('',(-38.,4.7,105.4));
#42231=CARTESIAN_POINT('',(37.9,4.7,100.3));
#42232=CARTESIAN_POINT('Origin',(-38.,4.7,105.4));
#42233=CARTESIAN_POINT('',(37.9,8.5,105.4));
#42234=CARTESIAN_POINT('',(-38.,8.5,105.4));
#42235=CARTESIAN_POINT('',(37.9,5.525,105.4));
#42236=CARTESIAN_POINT('Origin',(-38.,8.55,105.45));
#42237=CARTESIAN_POINT('',(-37.9,8.6,105.5));
#42238=CARTESIAN_POINT('',(-38.25,8.25,105.15));
#42239=CARTESIAN_POINT('',(37.9,8.6,105.5));
#42240=CARTESIAN_POINT('',(-38.,8.6,105.5));
#42241=CARTESIAN_POINT('',(37.95,8.55,105.45));
#42242=CARTESIAN_POINT('',(25.5833333333338,20.9166666666669,117.816666666666));
#42243=CARTESIAN_POINT('',(24.7875000000004,-4.61250000000026,92.2875000000004));
#42244=CARTESIAN_POINT('Origin',(-37.95,-5.225,105.95));
#42245=CARTESIAN_POINT('',(-37.95,-8.55,105.95));
#42246=CARTESIAN_POINT('',(-37.9,-8.5,106.));
#42247=CARTESIAN_POINT('',(-37.4041666666666,-8.00416666666666,106.495833333333));
#42248=CARTESIAN_POINT('',(-37.9,-4.2,106.));
#42249=CARTESIAN_POINT('',(-37.9,-5.225,106.));
#42250=CARTESIAN_POINT('',(-37.95,-4.15,105.95));
#42251=CARTESIAN_POINT('',(-37.7791666666667,-4.32083333333333,106.120833333333));
#42252=CARTESIAN_POINT('',(-38.,-4.2,105.9));
#42253=CARTESIAN_POINT('',(-39.1208333333333,-5.32083333333331,104.779166666667));
#42254=CARTESIAN_POINT('',(-38.,-8.5,105.9));
#42255=CARTESIAN_POINT('',(-38.,-5.225,105.9));
#42256=CARTESIAN_POINT('',(-38.8291666666667,-7.67083333333333,105.070833333333));
#42257=CARTESIAN_POINT('Origin',(-38.,-8.55,105.95));
#42258=CARTESIAN_POINT('',(-37.9,-8.6,105.9));
#42259=CARTESIAN_POINT('',(-37.6333333333333,-8.86666666666666,105.633333333333));
#42260=CARTESIAN_POINT('',(-25.7,-8.6,105.9));
#42261=CARTESIAN_POINT('',(-38.,-8.6,105.9));
#42262=CARTESIAN_POINT('',(-25.8,-8.5,106.));
#42263=CARTESIAN_POINT('',(-25.7,-8.6,105.9));
#42264=CARTESIAN_POINT('',(-38.,-8.5,106.));
#42265=CARTESIAN_POINT('Origin',(-37.95,-8.55,104.));
#42266=CARTESIAN_POINT('',(-38.,-8.5,105.5));
#42267=CARTESIAN_POINT('',(-38.,-8.5,104.));
#42268=CARTESIAN_POINT('',(-37.95,-8.55000000000001,105.45));
#42269=CARTESIAN_POINT('',(-37.8875,-8.61249999999999,105.3875));
#42270=CARTESIAN_POINT('',(-37.9,-8.6,105.5));
#42271=CARTESIAN_POINT('',(-38.2,-8.30000000000001,105.2));
#42272=CARTESIAN_POINT('',(-37.9,-8.6,104.));
#42273=CARTESIAN_POINT('Origin',(-38.,-6.35,102.));
#42274=CARTESIAN_POINT('',(-38.,-7.475,105.5));
#42275=CARTESIAN_POINT('',(-38.,-4.2,98.1));
#42276=CARTESIAN_POINT('',(-38.,-4.2,100.));
#42277=CARTESIAN_POINT('',(-38.,-8.5,98.1));
#42278=CARTESIAN_POINT('',(-38.,-7.475,98.1));
#42279=CARTESIAN_POINT('',(-38.,-8.5,100.3));
#42280=CARTESIAN_POINT('Origin',(-38.,-8.55,105.95));
#42281=CARTESIAN_POINT('',(25.7,-8.6,105.9));
#42282=CARTESIAN_POINT('',(37.9,-8.6,105.9));
#42283=CARTESIAN_POINT('',(-38.,-8.6,105.9));
#42284=CARTESIAN_POINT('',(37.95,-8.55000000000001,105.95));
#42285=CARTESIAN_POINT('',(24.9666666666671,-21.5333333333336,92.9666666666671));
#42286=CARTESIAN_POINT('',(37.9,-8.5,106.));
#42287=CARTESIAN_POINT('',(24.7375000000004,4.66250000000027,119.1625));
#42288=CARTESIAN_POINT('',(25.8,-8.5,106.));
#42289=CARTESIAN_POINT('',(-38.,-8.5,106.));
#42290=CARTESIAN_POINT('',(25.8,-8.5,106.));
#42291=CARTESIAN_POINT('Origin',(25.75,-8.55,106.));
#42292=CARTESIAN_POINT('',(25.8,-8.5,106.85));
#42293=CARTESIAN_POINT('',(25.8,-8.5,106.));
#42294=CARTESIAN_POINT('',(25.75,-8.55,106.9));
#42295=CARTESIAN_POINT('',(26.6,-7.70000000000001,106.05));
#42296=CARTESIAN_POINT('',(25.7,-8.6,106.85));
#42297=CARTESIAN_POINT('',(18.1500000000004,-16.1499999999998,99.2999999999999));
#42298=CARTESIAN_POINT('',(25.7,-8.6,106.));
#42299=CARTESIAN_POINT('Origin',(-38.,-8.6,106.));
#42300=CARTESIAN_POINT('',(-25.7,-8.6,106.85));
#42301=CARTESIAN_POINT('',(-19.,-8.6,106.85));
#42302=CARTESIAN_POINT('',(-25.7,-8.6,106.));
#42303=CARTESIAN_POINT('',(37.9,-8.6,105.5));
#42304=CARTESIAN_POINT('',(-38.,-8.6,105.5));
#42305=CARTESIAN_POINT('',(37.9,-8.6,104.));
#42306=CARTESIAN_POINT('Origin',(-19.,-8.525,106.925));
#42307=CARTESIAN_POINT('',(25.65,-8.45,107.));
#42308=CARTESIAN_POINT('',(25.65,-8.45,107.));
#42309=CARTESIAN_POINT('',(-25.65,-8.45,107.));
#42310=CARTESIAN_POINT('',(-19.,-8.45,107.));
#42311=CARTESIAN_POINT('',(-25.75,-8.55,106.9));
#42312=CARTESIAN_POINT('',(-25.65,-8.45,107.));
#42313=CARTESIAN_POINT('',(-24.4833333333334,-9.81666666666663,105.633333333333));
#42314=CARTESIAN_POINT('Origin',(25.725,-4.3,106.925));
#42315=CARTESIAN_POINT('',(25.8,8.5,106.85));
#42316=CARTESIAN_POINT('',(25.8,-4.3,106.85));
#42317=CARTESIAN_POINT('',(25.75,8.55,106.9));
#42318=CARTESIAN_POINT('',(28.0833333333333,6.21666666666668,104.566666666667));
#42319=CARTESIAN_POINT('',(25.65,8.45,107.));
#42320=CARTESIAN_POINT('',(25.65,8.45,107.));
#42321=CARTESIAN_POINT('',(25.65,-4.3,107.));
#42322=CARTESIAN_POINT('Origin',(-37.95,-7.475,105.45));
#42323=CARTESIAN_POINT('',(-37.9,-8.5,105.4));
#42324=CARTESIAN_POINT('',(-37.9,-7.475,105.4));
#42325=CARTESIAN_POINT('',(-37.7791666666667,-8.37916666666666,105.279166666667));
#42326=CARTESIAN_POINT('Origin',(-38.,-8.55,105.45));
#42327=CARTESIAN_POINT('',(37.9,-8.5,105.4));
#42328=CARTESIAN_POINT('',(-38.,-8.5,105.4));
#42329=CARTESIAN_POINT('',(37.95,-8.54999999999999,105.45));
#42330=CARTESIAN_POINT('',(25.1125000000005,4.28750000000024,92.6125000000005));
#42331=CARTESIAN_POINT('',(25.5333333333338,-20.9666666666669,117.866666666666));
#42332=CARTESIAN_POINT('Origin',(37.95,-8.55,104.));
#42333=CARTESIAN_POINT('',(38.,-8.5,105.5));
#42334=CARTESIAN_POINT('',(37.8875,-8.61249999999999,105.3875));
#42335=CARTESIAN_POINT('',(38.,-8.5,105.9));
#42336=CARTESIAN_POINT('',(38.,-8.5,104.));
#42337=CARTESIAN_POINT('',(38.8291666666667,-7.67083333333329,105.070833333333));
#42338=CARTESIAN_POINT('Origin',(37.95,-7.475,105.45));
#42339=CARTESIAN_POINT('',(37.9,-7.475,105.4));
#42340=CARTESIAN_POINT('',(38.,-4.6,105.5));
#42341=CARTESIAN_POINT('',(38.,-4.6,105.5));
#42342=CARTESIAN_POINT('',(38.,-7.475,105.5));
#42343=CARTESIAN_POINT('Origin',(-37.95,8.55,100.));
#42344=CARTESIAN_POINT('',(-37.9,8.6,98.1));
#42345=CARTESIAN_POINT('',(-37.9,8.6,100.));
#42346=CARTESIAN_POINT('',(-37.95,8.55000000000001,98.05));
#42347=CARTESIAN_POINT('',(-37.6333333333333,8.86666666666667,98.3666666666667));
#42348=CARTESIAN_POINT('',(-38.,8.5,98.1));
#42349=CARTESIAN_POINT('',(-38.8291666666667,7.67083333333329,98.9291666666667));
#42350=CARTESIAN_POINT('',(-38.,8.5,100.));
#42351=CARTESIAN_POINT('Origin',(-38.,8.6,98.));
#42352=CARTESIAN_POINT('',(37.9,8.6,98.1));
#42353=CARTESIAN_POINT('',(37.9,8.6,100.));
#42354=CARTESIAN_POINT('',(25.7,8.6,98.1));
#42355=CARTESIAN_POINT('',(-38.,8.6,98.1));
#42356=CARTESIAN_POINT('',(25.7,8.6,97.15));
#42357=CARTESIAN_POINT('',(25.7,8.6,97.5));
#42358=CARTESIAN_POINT('',(-25.7,8.6,97.15));
#42359=CARTESIAN_POINT('',(-19.,8.6,97.15));
#42360=CARTESIAN_POINT('',(-25.7,8.6,98.1));
#42361=CARTESIAN_POINT('',(-25.7,8.6,97.5));
#42362=CARTESIAN_POINT('',(-38.,8.6,98.1));
#42363=CARTESIAN_POINT('Origin',(-38.,8.55,98.05));
#42364=CARTESIAN_POINT('',(-25.8,8.5,98.));
#42365=CARTESIAN_POINT('',(-27.8833333333335,6.41666666666659,95.9166666666667));
#42366=CARTESIAN_POINT('',(-37.9,8.5,98.));
#42367=CARTESIAN_POINT('',(-38.,8.5,98.));
#42368=CARTESIAN_POINT('',(-37.4041666666667,8.00416666666663,97.5041666666666));
#42369=CARTESIAN_POINT('Origin',(-37.95,5.225,98.05));
#42370=CARTESIAN_POINT('',(-37.9,4.2,98.));
#42371=CARTESIAN_POINT('',(-37.9,5.225,98.));
#42372=CARTESIAN_POINT('',(-38.,4.2,98.1));
#42373=CARTESIAN_POINT('',(-37.9,4.2,98.));
#42374=CARTESIAN_POINT('',(-38.,5.225,98.1));
#42375=CARTESIAN_POINT('Origin',(-25.75,-8.55,106.));
#42376=CARTESIAN_POINT('',(-25.8,-8.5,106.85));
#42377=CARTESIAN_POINT('',(-28.0333333333333,-6.26666666666668,104.616666666667));
#42378=CARTESIAN_POINT('',(-25.8,-8.5,106.));
#42379=CARTESIAN_POINT('Origin',(-38.,-4.1,106.));
#42380=CARTESIAN_POINT('',(-25.8,-4.2,106.));
#42381=CARTESIAN_POINT('',(-25.8,2.25,106.));
#42382=CARTESIAN_POINT('',(-38.,-4.2,106.));
#42383=CARTESIAN_POINT('Origin',(-25.8,8.6,106.));
#42384=CARTESIAN_POINT('',(-25.8,8.5,106.85));
#42385=CARTESIAN_POINT('',(-25.8,4.3,106.85));
#42386=CARTESIAN_POINT('',(-25.8,8.5,106.));
#42387=CARTESIAN_POINT('',(-25.8,8.5,105.7));
#42388=CARTESIAN_POINT('',(-25.8,4.2,106.));
#42389=CARTESIAN_POINT('',(-25.8,8.6,106.));
#42390=CARTESIAN_POINT('',(-25.8,4.1,105.9));
#42391=CARTESIAN_POINT('',(-25.8,5.27500000000006,107.075));
#42392=CARTESIAN_POINT('',(-25.8,4.1,106.1));
#42393=CARTESIAN_POINT('',(-25.8,4.1,106.));
#42394=CARTESIAN_POINT('',(-25.8,-4.1,106.1));
#42395=CARTESIAN_POINT('',(-25.8,4.3,106.1));
#42396=CARTESIAN_POINT('',(-25.8,-4.1,105.9));
#42397=CARTESIAN_POINT('',(-25.8,-4.1,102.));
#42398=CARTESIAN_POINT('',(-25.8,-0.974999999999829,102.775));
#42399=CARTESIAN_POINT('Origin',(-25.725,4.3,106.925));
#42400=CARTESIAN_POINT('',(-25.65,8.45,107.));
#42401=CARTESIAN_POINT('',(-25.65,4.3,107.));
#42402=CARTESIAN_POINT('',(-25.75,8.55,106.9));
#42403=CARTESIAN_POINT('',(-25.65,8.45,107.));
#42404=CARTESIAN_POINT('',(-26.65,7.65000000000004,106.));
#42405=CARTESIAN_POINT('Origin',(-38.,4.2,98.1));
#42406=CARTESIAN_POINT('',(-37.9,4.1,98.1));
#42407=CARTESIAN_POINT('',(-37.9,4.1,98.1));
#42408=CARTESIAN_POINT('',(-38.,4.2,98.1));
#42409=CARTESIAN_POINT('Origin',(-37.95,4.15,104.));
#42410=CARTESIAN_POINT('',(-37.95,4.15,105.95));
#42411=CARTESIAN_POINT('',(-38.,4.2,105.9));
#42412=CARTESIAN_POINT('',(-38.8291666666667,5.02916666666671,105.070833333333));
#42413=CARTESIAN_POINT('',(-38.,4.2,104.));
#42414=CARTESIAN_POINT('',(-37.9,4.1,105.9));
#42415=CARTESIAN_POINT('',(-37.9,4.1,104.));
#42416=CARTESIAN_POINT('',(-37.6333333333333,3.83333333333332,105.633333333333));
#42417=CARTESIAN_POINT('Origin',(-38.,4.15,98.05));
#42418=CARTESIAN_POINT('',(-25.8,4.2,98.));
#42419=CARTESIAN_POINT('',(-25.8,4.1,98.1));
#42420=CARTESIAN_POINT('',(-25.8,5.52500000000006,96.675));
#42421=CARTESIAN_POINT('',(-38.,4.1,98.1));
#42422=CARTESIAN_POINT('',(-38.,4.2,98.));
#42423=CARTESIAN_POINT('Origin',(-38.,6.35,102.));
#42424=CARTESIAN_POINT('',(-38.,8.5,105.9));
#42425=CARTESIAN_POINT('',(-38.,7.475,105.9));
#42426=CARTESIAN_POINT('',(-38.,8.5,103.7));
#42427=CARTESIAN_POINT('Origin',(-37.95,7.475,105.95));
#42428=CARTESIAN_POINT('',(-37.9,4.2,106.));
#42429=CARTESIAN_POINT('',(-38.,4.1,105.9));
#42430=CARTESIAN_POINT('',(-37.9,8.5,106.));
#42431=CARTESIAN_POINT('',(-37.9,7.475,106.));
#42432=CARTESIAN_POINT('',(-37.95,8.55,105.95));
#42433=CARTESIAN_POINT('',(-37.7791666666667,8.37916666666665,106.120833333333));
#42434=CARTESIAN_POINT('',(-38.5041666666667,7.99583333333331,105.395833333333));
#42435=CARTESIAN_POINT('Origin',(-38.,4.15,105.95));
#42436=CARTESIAN_POINT('',(-38.,4.1,105.9));
#42437=CARTESIAN_POINT('',(-38.,4.2,106.));
#42438=CARTESIAN_POINT('Origin',(-38.,4.1,106.));
#42439=CARTESIAN_POINT('',(-25.8,4.1,97.9));
#42440=CARTESIAN_POINT('',(-25.8,4.1,101.5));
#42441=CARTESIAN_POINT('',(-25.7,4.1,98.));
#42442=CARTESIAN_POINT('',(-26.8000000000002,4.1,96.8999999999998));
#42443=CARTESIAN_POINT('',(25.7,4.1,98.));
#42444=CARTESIAN_POINT('',(-38.,4.1,98.));
#42445=CARTESIAN_POINT('',(25.8,4.1,97.9));
#42446=CARTESIAN_POINT('',(7.79999999999887,4.1,115.9));
#42447=CARTESIAN_POINT('',(25.8,4.1,98.1));
#42448=CARTESIAN_POINT('',(25.8,4.1,101.5));
#42449=CARTESIAN_POINT('',(37.9,4.1,98.1));
#42450=CARTESIAN_POINT('',(-38.,4.1,98.1));
#42451=CARTESIAN_POINT('',(37.9,4.1,105.9));
#42452=CARTESIAN_POINT('',(37.9,4.1,104.));
#42453=CARTESIAN_POINT('',(25.8,4.1,105.9));
#42454=CARTESIAN_POINT('',(-38.,4.1,105.9));
#42455=CARTESIAN_POINT('',(25.8,4.1,106.1));
#42456=CARTESIAN_POINT('',(25.8,4.1,106.));
#42457=CARTESIAN_POINT('',(25.7,4.1,106.));
#42458=CARTESIAN_POINT('',(9.79999999999887,4.1,90.1));
#42459=CARTESIAN_POINT('',(-25.7,4.1,106.));
#42460=CARTESIAN_POINT('',(-38.,4.1,106.));
#42461=CARTESIAN_POINT('',(-28.8000000000002,4.1,109.1));
#42462=CARTESIAN_POINT('Origin',(-38.,4.15,105.95));
#42463=CARTESIAN_POINT('',(37.95,4.15,105.95));
#42464=CARTESIAN_POINT('',(37.9,4.2,106.));
#42465=CARTESIAN_POINT('',(24.7375000000004,17.3625000000003,119.1625));
#42466=CARTESIAN_POINT('',(25.8,4.2,106.));
#42467=CARTESIAN_POINT('',(-38.,4.2,106.));
#42468=CARTESIAN_POINT('',(25.8,0.974999999999829,102.775));
#42469=CARTESIAN_POINT('',(24.9666666666671,-8.83333333333357,92.9666666666671));
#42470=CARTESIAN_POINT('Origin',(37.95,7.475,105.95));
#42471=CARTESIAN_POINT('',(38.,4.2,105.9));
#42472=CARTESIAN_POINT('',(38.,4.2,105.9));
#42473=CARTESIAN_POINT('',(38.,8.5,105.9));
#42474=CARTESIAN_POINT('',(38.,7.475,105.9));
#42475=CARTESIAN_POINT('',(37.95,8.55,105.95));
#42476=CARTESIAN_POINT('',(38.5041666666667,7.99583333333331,105.395833333333));
#42477=CARTESIAN_POINT('',(37.9,8.5,106.));
#42478=CARTESIAN_POINT('',(25.1125000000004,-4.28750000000023,118.7875));
#42479=CARTESIAN_POINT('',(37.9,7.475,106.));
#42480=CARTESIAN_POINT('Origin',(37.95,4.15,104.));
#42481=CARTESIAN_POINT('',(37.95,4.15,98.05));
#42482=CARTESIAN_POINT('',(24.3000000000005,-9.50000000000025,111.7));
#42483=CARTESIAN_POINT('',(38.,4.2,98.1));
#42484=CARTESIAN_POINT('',(38.,4.2,98.1));
#42485=CARTESIAN_POINT('',(38.,4.2,104.));
#42486=CARTESIAN_POINT('Origin',(-38.,8.55,98.05));
#42487=CARTESIAN_POINT('',(37.95,8.55000000000001,98.05));
#42488=CARTESIAN_POINT('',(24.9666666666671,21.5333333333336,111.033333333333));
#42489=CARTESIAN_POINT('',(37.9,8.5,98.));
#42490=CARTESIAN_POINT('',(24.7375000000004,-4.66250000000027,84.8375000000004));
#42491=CARTESIAN_POINT('',(25.8,8.5,98.));
#42492=CARTESIAN_POINT('',(-38.,8.5,98.));
#42493=CARTESIAN_POINT('',(25.8,8.5,98.));
#42494=CARTESIAN_POINT('Origin',(25.75,8.55,97.5));
#42495=CARTESIAN_POINT('',(25.8,8.5,97.15));
#42496=CARTESIAN_POINT('',(25.8,8.5,97.5));
#42497=CARTESIAN_POINT('',(25.75,8.55,97.1));
#42498=CARTESIAN_POINT('',(27.9499999999999,6.35000000000002,99.3000000000001));
#42499=CARTESIAN_POINT('',(18.2333333333337,16.0666666666664,104.616666666667));
#42500=CARTESIAN_POINT('Origin',(37.95,8.55,100.));
#42501=CARTESIAN_POINT('',(38.,8.5,98.5));
#42502=CARTESIAN_POINT('',(37.8875,8.61249999999999,98.6125));
#42503=CARTESIAN_POINT('',(38.,8.5,98.1));
#42504=CARTESIAN_POINT('',(38.,8.5,100.));
#42505=CARTESIAN_POINT('',(38.8291666666667,7.67083333333329,98.9291666666667));
#42506=CARTESIAN_POINT('Origin',(-19.,8.525,97.075));
#42507=CARTESIAN_POINT('',(25.65,8.45,97.));
#42508=CARTESIAN_POINT('',(25.65,8.45,97.));
#42509=CARTESIAN_POINT('',(-25.65,8.45,97.));
#42510=CARTESIAN_POINT('',(-19.,8.45,97.));
#42511=CARTESIAN_POINT('',(-25.75,8.55,97.1));
#42512=CARTESIAN_POINT('',(-25.8,8.6,97.15));
#42513=CARTESIAN_POINT('',(-24.5666666666667,9.73333333333331,98.2833333333334));
#42514=CARTESIAN_POINT('Origin',(25.75,-4.3,97.95));
#42515=CARTESIAN_POINT('',(25.7,-4.1,98.));
#42516=CARTESIAN_POINT('',(25.8,-4.1,97.9));
#42517=CARTESIAN_POINT('',(9.79999999999887,-4.1,113.9));
#42518=CARTESIAN_POINT('',(25.8,-4.3,97.9));
#42519=CARTESIAN_POINT('',(25.7,-4.3,98.));
#42520=CARTESIAN_POINT('Origin',(25.8,-8.6,97.));
#42521=CARTESIAN_POINT('',(25.8,4.2,98.));
#42522=CARTESIAN_POINT('',(25.8,-2.25,98.));
#42523=CARTESIAN_POINT('',(25.8,1.22499999999983,100.975));
#42524=CARTESIAN_POINT('',(25.8,-4.1,98.1));
#42525=CARTESIAN_POINT('',(25.8,-4.1,97.5));
#42526=CARTESIAN_POINT('',(25.8,-4.2,98.));
#42527=CARTESIAN_POINT('',(25.8,-5.52500000000006,96.675));
#42528=CARTESIAN_POINT('',(25.8,-8.5,98.));
#42529=CARTESIAN_POINT('',(25.8,-8.6,98.));
#42530=CARTESIAN_POINT('',(25.8,-8.5,97.15));
#42531=CARTESIAN_POINT('',(25.8,-8.5,97.8));
#42532=CARTESIAN_POINT('',(25.8,-4.3,97.15));
#42533=CARTESIAN_POINT('Origin',(-38.,4.15,98.05));
#42534=CARTESIAN_POINT('',(37.9,4.2,98.));
#42535=CARTESIAN_POINT('',(-38.,4.2,98.));
#42536=CARTESIAN_POINT('',(25.1125000000005,16.9875000000002,85.2125000000004));
#42537=CARTESIAN_POINT('Origin',(37.95,5.225,98.05));
#42538=CARTESIAN_POINT('',(38.,5.225,98.1));
#42539=CARTESIAN_POINT('',(37.9,5.225,98.));
#42540=CARTESIAN_POINT('Origin',(37.95,5.525,105.45));
#42541=CARTESIAN_POINT('',(38.,8.5,105.5));
#42542=CARTESIAN_POINT('',(38.1625,8.33749999999997,105.6625));
#42543=CARTESIAN_POINT('',(38.,4.6,105.5));
#42544=CARTESIAN_POINT('',(38.,5.525,105.5));
#42545=CARTESIAN_POINT('',(38.,4.6,105.5));
#42546=CARTESIAN_POINT('Origin',(37.95,4.65,100.3));
#42547=CARTESIAN_POINT('',(38.,4.6,98.5));
#42548=CARTESIAN_POINT('',(38.,4.6,100.3));
#42549=CARTESIAN_POINT('',(38.,4.6,98.5));
#42550=CARTESIAN_POINT('Origin',(37.95,7.475,98.55));
#42551=CARTESIAN_POINT('',(38.,7.475,98.5));
#42552=CARTESIAN_POINT('Origin',(38.,6.35,102.));
#42553=CARTESIAN_POINT('',(38.,8.5,103.7));
#42554=CARTESIAN_POINT('Origin',(37.95,8.55,103.7));
#42555=CARTESIAN_POINT('',(37.9,8.6,105.9));
#42556=CARTESIAN_POINT('',(37.9,8.6,103.7));
#42557=CARTESIAN_POINT('',(24.9166666666671,21.5833333333336,92.9166666666671));
#42558=CARTESIAN_POINT('Origin',(-38.,4.1,98.));
#42559=CARTESIAN_POINT('Origin',(-38.,8.6,106.));
#42560=CARTESIAN_POINT('',(25.8,8.5,106.));
#42561=CARTESIAN_POINT('',(-38.,8.5,106.));
#42562=CARTESIAN_POINT('',(25.8,0.,106.));
#42563=CARTESIAN_POINT('Origin',(-38.,8.55,105.95));
#42564=CARTESIAN_POINT('',(25.7,8.6,105.9));
#42565=CARTESIAN_POINT('',(-38.,8.6,105.9));
#42566=CARTESIAN_POINT('',(25.7,8.6,105.9));
#42567=CARTESIAN_POINT('Origin',(-38.,8.6,105.4));
#42568=CARTESIAN_POINT('',(-37.9,8.6,105.9));
#42569=CARTESIAN_POINT('',(-37.9,8.6,103.7));
#42570=CARTESIAN_POINT('',(-25.7,8.6,105.9));
#42571=CARTESIAN_POINT('',(-38.,8.6,105.9));
#42572=CARTESIAN_POINT('',(-25.7,8.6,106.85));
#42573=CARTESIAN_POINT('',(-25.7,8.6,105.7));
#42574=CARTESIAN_POINT('',(25.7,8.6,106.85));
#42575=CARTESIAN_POINT('',(-19.,8.6,106.85));
#42576=CARTESIAN_POINT('',(25.7,8.6,105.7));
#42577=CARTESIAN_POINT('Origin',(25.75,8.55,105.7));
#42578=CARTESIAN_POINT('',(18.1000000000004,16.1999999999998,99.2499999999999));
#42579=CARTESIAN_POINT('',(25.8,8.5,105.7));
#42580=CARTESIAN_POINT('Origin',(-19.,8.525,106.925));
#42581=CARTESIAN_POINT('',(-24.4333333333333,9.86666666666665,105.583333333333));
#42582=CARTESIAN_POINT('',(-19.,8.45,107.));
#42583=CARTESIAN_POINT('Origin',(-25.75,8.55,105.7));
#42584=CARTESIAN_POINT('',(-25.7,8.6,105.9));
#42585=CARTESIAN_POINT('Origin',(-38.,8.55,105.95));
#42586=CARTESIAN_POINT('',(-37.5833333333333,8.91666666666667,105.583333333333));
#42587=CARTESIAN_POINT('',(-38.,8.5,106.));
#42588=CARTESIAN_POINT('Origin',(-38.,8.6,106.));
#42589=CARTESIAN_POINT('Origin',(-25.75,8.55,97.5));
#42590=CARTESIAN_POINT('',(-25.8,8.5,97.15));
#42591=CARTESIAN_POINT('',(-26.5166666666666,7.78333333333337,97.8666666666667));
#42592=CARTESIAN_POINT('',(-25.8,8.5,97.5));
#42593=CARTESIAN_POINT('Origin',(-25.75,4.3,97.95));
#42594=CARTESIAN_POINT('',(-25.8,-4.1,97.9));
#42595=CARTESIAN_POINT('',(-25.8,4.3,97.9));
#42596=CARTESIAN_POINT('',(-25.7,-4.1,98.));
#42597=CARTESIAN_POINT('',(-28.8000000000002,-4.1,94.9));
#42598=CARTESIAN_POINT('',(-25.7,4.3,98.));
#42599=CARTESIAN_POINT('Origin',(-25.8,8.6,97.));
#42600=CARTESIAN_POINT('',(-25.8,-8.5,97.15));
#42601=CARTESIAN_POINT('',(-25.8,4.3,97.15));
#42602=CARTESIAN_POINT('',(-25.8,-8.5,98.));
#42603=CARTESIAN_POINT('',(-25.8,-8.5,97.8));
#42604=CARTESIAN_POINT('',(-25.8,-4.2,98.));
#42605=CARTESIAN_POINT('',(-25.8,0.,98.));
#42606=CARTESIAN_POINT('',(-25.8,-4.1,98.1));
#42607=CARTESIAN_POINT('',(-25.8,-1.22499999999983,100.975));
#42608=CARTESIAN_POINT('',(-25.8,-4.1,97.5));
#42609=CARTESIAN_POINT('',(-25.8,6.35,98.));
#42610=CARTESIAN_POINT('Origin',(25.75,-4.3,106.05));
#42611=CARTESIAN_POINT('',(25.8,-4.1,106.1));
#42612=CARTESIAN_POINT('',(25.8,-4.3,106.1));
#42613=CARTESIAN_POINT('',(25.7,-4.1,106.));
#42614=CARTESIAN_POINT('',(7.79999999999887,-4.1,88.1000000000002));
#42615=CARTESIAN_POINT('',(25.7,-4.3,106.));
#42616=CARTESIAN_POINT('Origin',(0.,0.,106.));
#42617=CARTESIAN_POINT('',(-25.7,-4.1,106.));
#42618=CARTESIAN_POINT('',(-38.,-4.1,106.));
#42619=CARTESIAN_POINT('',(-25.7,4.3,106.));
#42620=CARTESIAN_POINT('',(-19.105,7.40911313484149E-17,106.));
#42621=CARTESIAN_POINT('Origin',(-18.5,0.,106.));
#42622=CARTESIAN_POINT('',(17.895,7.40911313484149E-17,106.));
#42623=CARTESIAN_POINT('Origin',(18.5,0.,106.));
#42624=CARTESIAN_POINT('Origin',(-38.,-4.15,105.95));
#42625=CARTESIAN_POINT('',(37.95,-4.15,105.95));
#42626=CARTESIAN_POINT('',(37.9,-4.1,105.9));
#42627=CARTESIAN_POINT('',(24.3000000000005,9.50000000000025,92.3000000000005));
#42628=CARTESIAN_POINT('',(25.8,-4.1,105.9));
#42629=CARTESIAN_POINT('',(-38.,-4.1,105.9));
#42630=CARTESIAN_POINT('',(25.8,-4.2,106.));
#42631=CARTESIAN_POINT('',(25.8,-5.27500000000006,107.075));
#42632=CARTESIAN_POINT('',(37.9,-4.2,106.));
#42633=CARTESIAN_POINT('',(-38.,-4.2,106.));
#42634=CARTESIAN_POINT('',(25.1125000000005,-16.9875000000002,118.7875));
#42635=CARTESIAN_POINT('Origin',(-38.,-4.1,98.));
#42636=CARTESIAN_POINT('',(25.8,-4.1,102.));
#42637=CARTESIAN_POINT('',(37.9,-4.1,98.1));
#42638=CARTESIAN_POINT('',(37.9,-4.1,100.));
#42639=CARTESIAN_POINT('',(-38.,-4.1,98.1));
#42640=CARTESIAN_POINT('',(-38.,-4.1,98.));
#42641=CARTESIAN_POINT('',(-37.9,-4.1,98.1));
#42642=CARTESIAN_POINT('',(-38.,-4.1,98.1));
#42643=CARTESIAN_POINT('',(-37.9,-4.1,105.9));
#42644=CARTESIAN_POINT('',(-37.9,-4.1,100.));
#42645=CARTESIAN_POINT('',(-38.,-4.1,105.9));
#42646=CARTESIAN_POINT('',(-26.8000000000002,-4.1,107.1));
#42647=CARTESIAN_POINT('Origin',(37.95,-4.15,100.));
#42648=CARTESIAN_POINT('',(38.,-4.2,105.9));
#42649=CARTESIAN_POINT('',(38.,-4.2,105.9));
#42650=CARTESIAN_POINT('',(38.,-4.2,98.1));
#42651=CARTESIAN_POINT('',(38.,-4.2,100.));
#42652=CARTESIAN_POINT('',(38.,-4.2,98.1));
#42653=CARTESIAN_POINT('Origin',(37.95,-5.225,105.95));
#42654=CARTESIAN_POINT('',(38.,-5.225,105.9));
#42655=CARTESIAN_POINT('',(37.9,-5.225,106.));
#42656=CARTESIAN_POINT('Origin',(-37.95,8.55,103.7));
#42657=CARTESIAN_POINT('Origin',(-25.75,4.3,106.05));
#42658=CARTESIAN_POINT('Origin',(-37.95,-4.15,100.));
#42659=CARTESIAN_POINT('',(-38.,-4.2,106.));
#42660=CARTESIAN_POINT('',(-37.95,-4.15,98.05));
#42661=CARTESIAN_POINT('',(-37.6333333333333,-3.83333333333334,98.3666666666666));
#42662=CARTESIAN_POINT('',(-38.8291666666667,-5.02916666666667,98.9291666666666));
#42663=CARTESIAN_POINT('Origin',(-38.,-4.15,105.95));
#42664=CARTESIAN_POINT('Origin',(-38.,-4.15,98.05));
#42665=CARTESIAN_POINT('',(-37.9,-4.2,98.));
#42666=CARTESIAN_POINT('',(-38.,-4.2,98.));
#42667=CARTESIAN_POINT('',(-38.,-4.1,98.1));
#42668=CARTESIAN_POINT('Origin',(37.95,-5.525,98.55));
#42669=CARTESIAN_POINT('',(38.,-8.5,98.5));
#42670=CARTESIAN_POINT('',(38.1625,-8.33749999999997,98.3375));
#42671=CARTESIAN_POINT('',(38.,-4.6,98.5));
#42672=CARTESIAN_POINT('',(38.,-5.525,98.5));
#42673=CARTESIAN_POINT('',(38.,-4.6,98.5));
#42674=CARTESIAN_POINT('Origin',(37.95,-4.65,103.7));
#42675=CARTESIAN_POINT('',(38.,-4.6,103.7));
#42676=CARTESIAN_POINT('Origin',(38.,-6.35,102.));
#42677=CARTESIAN_POINT('',(38.,-8.5,98.1));
#42678=CARTESIAN_POINT('',(38.,-8.5,100.3));
#42679=CARTESIAN_POINT('',(38.,-7.475,98.1));
#42680=CARTESIAN_POINT('Origin',(37.95,-8.55,100.3));
#42681=CARTESIAN_POINT('',(37.9,-8.6,98.1));
#42682=CARTESIAN_POINT('',(37.9,-8.6,100.3));
#42683=CARTESIAN_POINT('',(37.95,-8.55,98.05));
#42684=CARTESIAN_POINT('',(24.9166666666671,-21.5833333333336,111.083333333333));
#42685=CARTESIAN_POINT('',(38.5041666666667,-7.99583333333331,98.6041666666667));
#42686=CARTESIAN_POINT('Origin',(37.9,-4.1,98.1));
#42687=CARTESIAN_POINT('',(37.9,-4.2,98.));
#42688=CARTESIAN_POINT('',(37.9,-4.2,98.));
#42689=CARTESIAN_POINT('',(37.9,-4.1,98.1));
#42690=CARTESIAN_POINT('Origin',(-38.,-4.15,98.05));
#42691=CARTESIAN_POINT('',(-38.,-4.2,98.));
#42692=CARTESIAN_POINT('Origin',(37.95,-7.475,98.05));
#42693=CARTESIAN_POINT('',(37.9,-8.5,98.));
#42694=CARTESIAN_POINT('',(25.1125000000004,4.28750000000023,85.2125000000004));
#42695=CARTESIAN_POINT('',(37.9,-7.475,98.));
#42696=CARTESIAN_POINT('Origin',(-38.,-8.6,98.));
#42697=CARTESIAN_POINT('',(-38.,-8.5,98.));
#42698=CARTESIAN_POINT('Origin',(-38.,-8.55,98.05));
#42699=CARTESIAN_POINT('',(25.7,-8.6,98.1));
#42700=CARTESIAN_POINT('',(-38.,-8.6,98.1));
#42701=CARTESIAN_POINT('',(25.7,-8.6,98.1));
#42702=CARTESIAN_POINT('Origin',(-37.95,-7.475,98.05));
#42703=CARTESIAN_POINT('',(-37.9,-8.5,98.));
#42704=CARTESIAN_POINT('',(-37.9,-7.475,98.));
#42705=CARTESIAN_POINT('',(-37.95,-8.55,98.05));
#42706=CARTESIAN_POINT('',(-37.7791666666667,-8.37916666666666,97.8791666666667));
#42707=CARTESIAN_POINT('',(-38.5041666666667,-7.99583333333334,98.6041666666666));
#42708=CARTESIAN_POINT('Origin',(-38.,-8.55,98.05));
#42709=CARTESIAN_POINT('',(-38.,-8.5,98.));
#42710=CARTESIAN_POINT('',(-25.7,-8.6,98.1));
#42711=CARTESIAN_POINT('',(-25.7,-8.6,98.1));
#42712=CARTESIAN_POINT('',(-37.9,-8.6,98.1));
#42713=CARTESIAN_POINT('',(-38.,-8.6,98.1));
#42714=CARTESIAN_POINT('',(-37.5833333333333,-8.91666666666666,98.4166666666666));
#42715=CARTESIAN_POINT('Origin',(-38.,-8.6,98.));
#42716=CARTESIAN_POINT('Origin',(-38.,-8.6,98.6));
#42717=CARTESIAN_POINT('',(-37.9,-8.6,100.3));
#42718=CARTESIAN_POINT('',(-25.7,-8.6,97.15));
#42719=CARTESIAN_POINT('',(-25.7,-8.6,97.8));
#42720=CARTESIAN_POINT('',(25.7,-8.6,97.15));
#42721=CARTESIAN_POINT('',(-19.,-8.6,97.15));
#42722=CARTESIAN_POINT('',(25.7,-8.6,97.8));
#42723=CARTESIAN_POINT('Origin',(25.75,-8.55,97.8));
#42724=CARTESIAN_POINT('',(25.75,-8.55,97.1));
#42725=CARTESIAN_POINT('',(18.1833333333337,-16.1166666666664,104.666666666667));
#42726=CARTESIAN_POINT('',(26.5666666666666,-7.73333333333334,97.9166666666667));
#42727=CARTESIAN_POINT('Origin',(25.725,-4.3,97.075));
#42728=CARTESIAN_POINT('',(25.65,-8.45,97.));
#42729=CARTESIAN_POINT('',(25.65,-8.45,97.));
#42730=CARTESIAN_POINT('',(25.65,-4.3,97.));
#42731=CARTESIAN_POINT('Origin',(-19.,-8.525,97.075));
#42732=CARTESIAN_POINT('',(-25.75,-8.55,97.1));
#42733=CARTESIAN_POINT('',(-24.5166666666667,-9.7833333333333,98.3333333333333));
#42734=CARTESIAN_POINT('',(-25.65,-8.45,97.));
#42735=CARTESIAN_POINT('',(-25.65,-8.45,97.));
#42736=CARTESIAN_POINT('',(-19.,-8.45,97.));
#42737=CARTESIAN_POINT('Origin',(-25.75,-8.55,97.8));
#42738=CARTESIAN_POINT('',(-27.9999999999999,-6.30000000000002,99.3500000000001));
#42739=CARTESIAN_POINT('Origin',(-25.725,4.3,97.075));
#42740=CARTESIAN_POINT('',(-25.65,4.3,97.));
#42741=CARTESIAN_POINT('Origin',(-37.95,-8.55,100.3));
#42742=CARTESIAN_POINT('Origin',(0.,-7.4375534806121E-17,91.2146446609407));
#42743=CARTESIAN_POINT('',(2.5,-3.06161699786838E-16,91.3));
#42744=CARTESIAN_POINT('',(-2.5,-3.06161699786838E-16,91.3));
#42745=CARTESIAN_POINT('Origin',(0.,0.,91.3));
#42746=CARTESIAN_POINT('Origin',(0.,0.,91.3));
#42747=CARTESIAN_POINT('',(2.42928932188135,2.97502139224484E-16,91.1292893218813));
#42748=CARTESIAN_POINT('',(2.46464466094067,3.01831919505661E-16,91.2146446609407));
#42749=CARTESIAN_POINT('',(-2.42928932188135,-2.97502139224484E-16,91.1292893218813));
#42750=CARTESIAN_POINT('Origin',(0.,-1.48751069612242E-16,91.1292893218813));
#42751=CARTESIAN_POINT('Origin',(0.,-1.48751069612242E-16,91.1292893218813));
#42752=CARTESIAN_POINT('Origin',(0.,0.,91.1));
#42753=CARTESIAN_POINT('',(-2.37071067811866,-2.90328324366247E-16,91.0707106781187));
#42754=CARTESIAN_POINT('',(-2.4,-2.93915231795365E-16,91.1));
#42755=CARTESIAN_POINT('',(2.37071067811866,-2.90328324366247E-16,91.0707106781187));
#42756=CARTESIAN_POINT('Origin',(0.,-1.45164162183123E-16,91.0707106781187));
#42757=CARTESIAN_POINT('Origin',(0.,-1.45164162183123E-16,91.0707106781187));
#42758=CARTESIAN_POINT('Origin',(0.,0.,93.95));
#42759=CARTESIAN_POINT('',(-2.5,-3.06161699786838E-16,96.7));
#42760=CARTESIAN_POINT('Origin',(0.,0.,96.7));
#42761=CARTESIAN_POINT('',(-2.5,-3.06161699786838E-16,93.95));
#42762=CARTESIAN_POINT('Origin',(0.,-7.25820810915617E-17,91.0353553390593));
#42763=CARTESIAN_POINT('',(2.2,2.69422295812418E-16,91.));
#42764=CARTESIAN_POINT('',(2.28535533905933,2.79875310089332E-16,91.0353553390593));
#42765=CARTESIAN_POINT('Origin',(0.,0.,91.));
#42766=CARTESIAN_POINT('Origin',(2.3,0.,91.));
#42767=CARTESIAN_POINT('Origin',(18.5,0.,106.05));
#42768=CARTESIAN_POINT('',(17.995,-6.18446633569412E-17,106.1));
#42769=CARTESIAN_POINT('',(17.945,6.79678973526781E-17,106.05));
#42770=CARTESIAN_POINT('Origin',(18.5,0.,106.1));
#42771=CARTESIAN_POINT('Origin',(18.5,0.,106.));
#42772=CARTESIAN_POINT('',(17.995,6.18446633569412E-17,106.9));
#42773=CARTESIAN_POINT('',(17.995,-6.18446633569412E-17,106.));
#42774=CARTESIAN_POINT('Origin',(18.5,0.,106.9));
#42775=CARTESIAN_POINT('Origin',(18.5,0.,106.95));
#42776=CARTESIAN_POINT('',(17.895,-7.40911313484149E-17,107.));
#42777=CARTESIAN_POINT('Origin',(18.5,0.,107.));
#42778=CARTESIAN_POINT('',(17.945,-6.79678973526781E-17,106.95));
#42779=CARTESIAN_POINT('Origin',(0.,0.,107.));
#42780=CARTESIAN_POINT('',(-19.105,-7.40911313484149E-17,107.));
#42781=CARTESIAN_POINT('Origin',(-18.5,0.,107.));
#42782=CARTESIAN_POINT('Origin',(-18.5,0.,106.05));
#42783=CARTESIAN_POINT('',(-19.005,-6.18446633569412E-17,106.1));
#42784=CARTESIAN_POINT('',(-19.055,6.79678973526781E-17,106.05));
#42785=CARTESIAN_POINT('Origin',(-18.5,0.,106.1));
#42786=CARTESIAN_POINT('Origin',(-18.5,0.,106.));
#42787=CARTESIAN_POINT('',(-19.005,6.18446633569412E-17,106.9));
#42788=CARTESIAN_POINT('',(-19.005,-6.18446633569412E-17,106.));
#42789=CARTESIAN_POINT('Origin',(-18.5,0.,106.9));
#42790=CARTESIAN_POINT('Origin',(-18.5,0.,106.95));
#42791=CARTESIAN_POINT('',(-19.055,-6.79678973526781E-17,106.95));
#42792=CARTESIAN_POINT('Origin',(0.,0.,96.875));
#42793=CARTESIAN_POINT('',(-2.75714285714286,-3.37652617479199E-16,97.));
#42794=CARTESIAN_POINT('Origin',(0.,0.,97.));
#42795=CARTESIAN_POINT('',(-2.65,-3.24531401774049E-16,96.875));
#42796=CARTESIAN_POINT('Origin',(-38.,-8.6,105.4));
#42797=CARTESIAN_POINT('Origin',(-38.,4.1,98.));
#42798=CARTESIAN_POINT('Origin',(0.,0.,97.));
#42799=CARTESIAN_POINT('Origin',(0.,0.,98.));
#42800=CARTESIAN_POINT('Origin',(25.8,-8.6,106.));
#42801=CARTESIAN_POINT('',(25.8,-6.35,106.));
#42802=CARTESIAN_POINT('Origin',(-38.,-4.1,106.));
#71453=UNCERTAINTY_MEASURE_WITH_UNIT(LENGTH_MEASURE(0.001),#71493,
'DISTANCE_ACCURACY_VALUE',
'Maximum model space distance between geometric entities at asserted c
onnectivities');
#71471=UNCERTAINTY_MEASURE_WITH_UNIT(LENGTH_MEASURE(0.001),#71493,
'DISTANCE_ACCURACY_VALUE',
'Maximum model space distance between geometric entities at asserted c
onnectivities');
#71474=(
GEOMETRIC_REPRESENTATION_CONTEXT(3)
GLOBAL_UNCERTAINTY_ASSIGNED_CONTEXT((#71453))
GLOBAL_UNIT_ASSIGNED_CONTEXT((#71493,#71495,#71496))
REPRESENTATION_CONTEXT('','3D')
);
#71492=(
GEOMETRIC_REPRESENTATION_CONTEXT(3)
GLOBAL_UNCERTAINTY_ASSIGNED_CONTEXT((#71471))
GLOBAL_UNIT_ASSIGNED_CONTEXT((#71493,#71495,#71496))
REPRESENTATION_CONTEXT('','3D')
);
#71493=(
LENGTH_UNIT()
NAMED_UNIT(*)
SI_UNIT(.CENTI.,.METRE.)
);
#71495=(
NAMED_UNIT(*)
PLANE_ANGLE_UNIT()
SI_UNIT($,.RADIAN.)
);
#71496=(
NAMED_UNIT(*)
SI_UNIT($,.STERADIAN.)
SOLID_ANGLE_UNIT()
);
#71499=SHAPE_DEFINITION_REPRESENTATION(#71519,#71604);
#71519=PRODUCT_DEFINITION_SHAPE('',$,#71625);
#71604=SHAPE_REPRESENTATION('',(#29045),#71474);
#71622=PRODUCT_DEFINITION_CONTEXT('part definition',#71684,'design');
#71625=PRODUCT_DEFINITION('2026-10-19-03-21-49-945',
'03_Movable_Press_Platen_Twin_C80_Shaft_D50',#71645,#71622);
#71645=PRODUCT_DEFINITION_FORMATION('',$,#71688);
#71684=APPLICATION_CONTEXT(
'Core Data for Automotive Mechanical Design Process');
#71685=PRODUCT_CONTEXT('part definition',#71684,'mechanical');
#71688=PRODUCT('2026-10-19-03-21-49-945',
'03_Movable_Press_Platen_Twin_C80_Shaft_D50',$,(#71685));
#71881=COLOUR_RGB('Grey',0.48,0.52,0.57);
#71882=FILL_AREA_STYLE_COLOUR('',#71881);
#71883=FILL_AREA_STYLE('',(#71882));
#71884=SURFACE_STYLE_FILL_AREA(#71883);
#71885=SURFACE_SIDE_STYLE('',(#71884));
#71886=SURFACE_STYLE_USAGE(.BOTH.,#71885);
#71887=PRESENTATION_STYLE_ASSIGNMENT((#71886));
ENDSEC;
END-ISO-10303-21;
